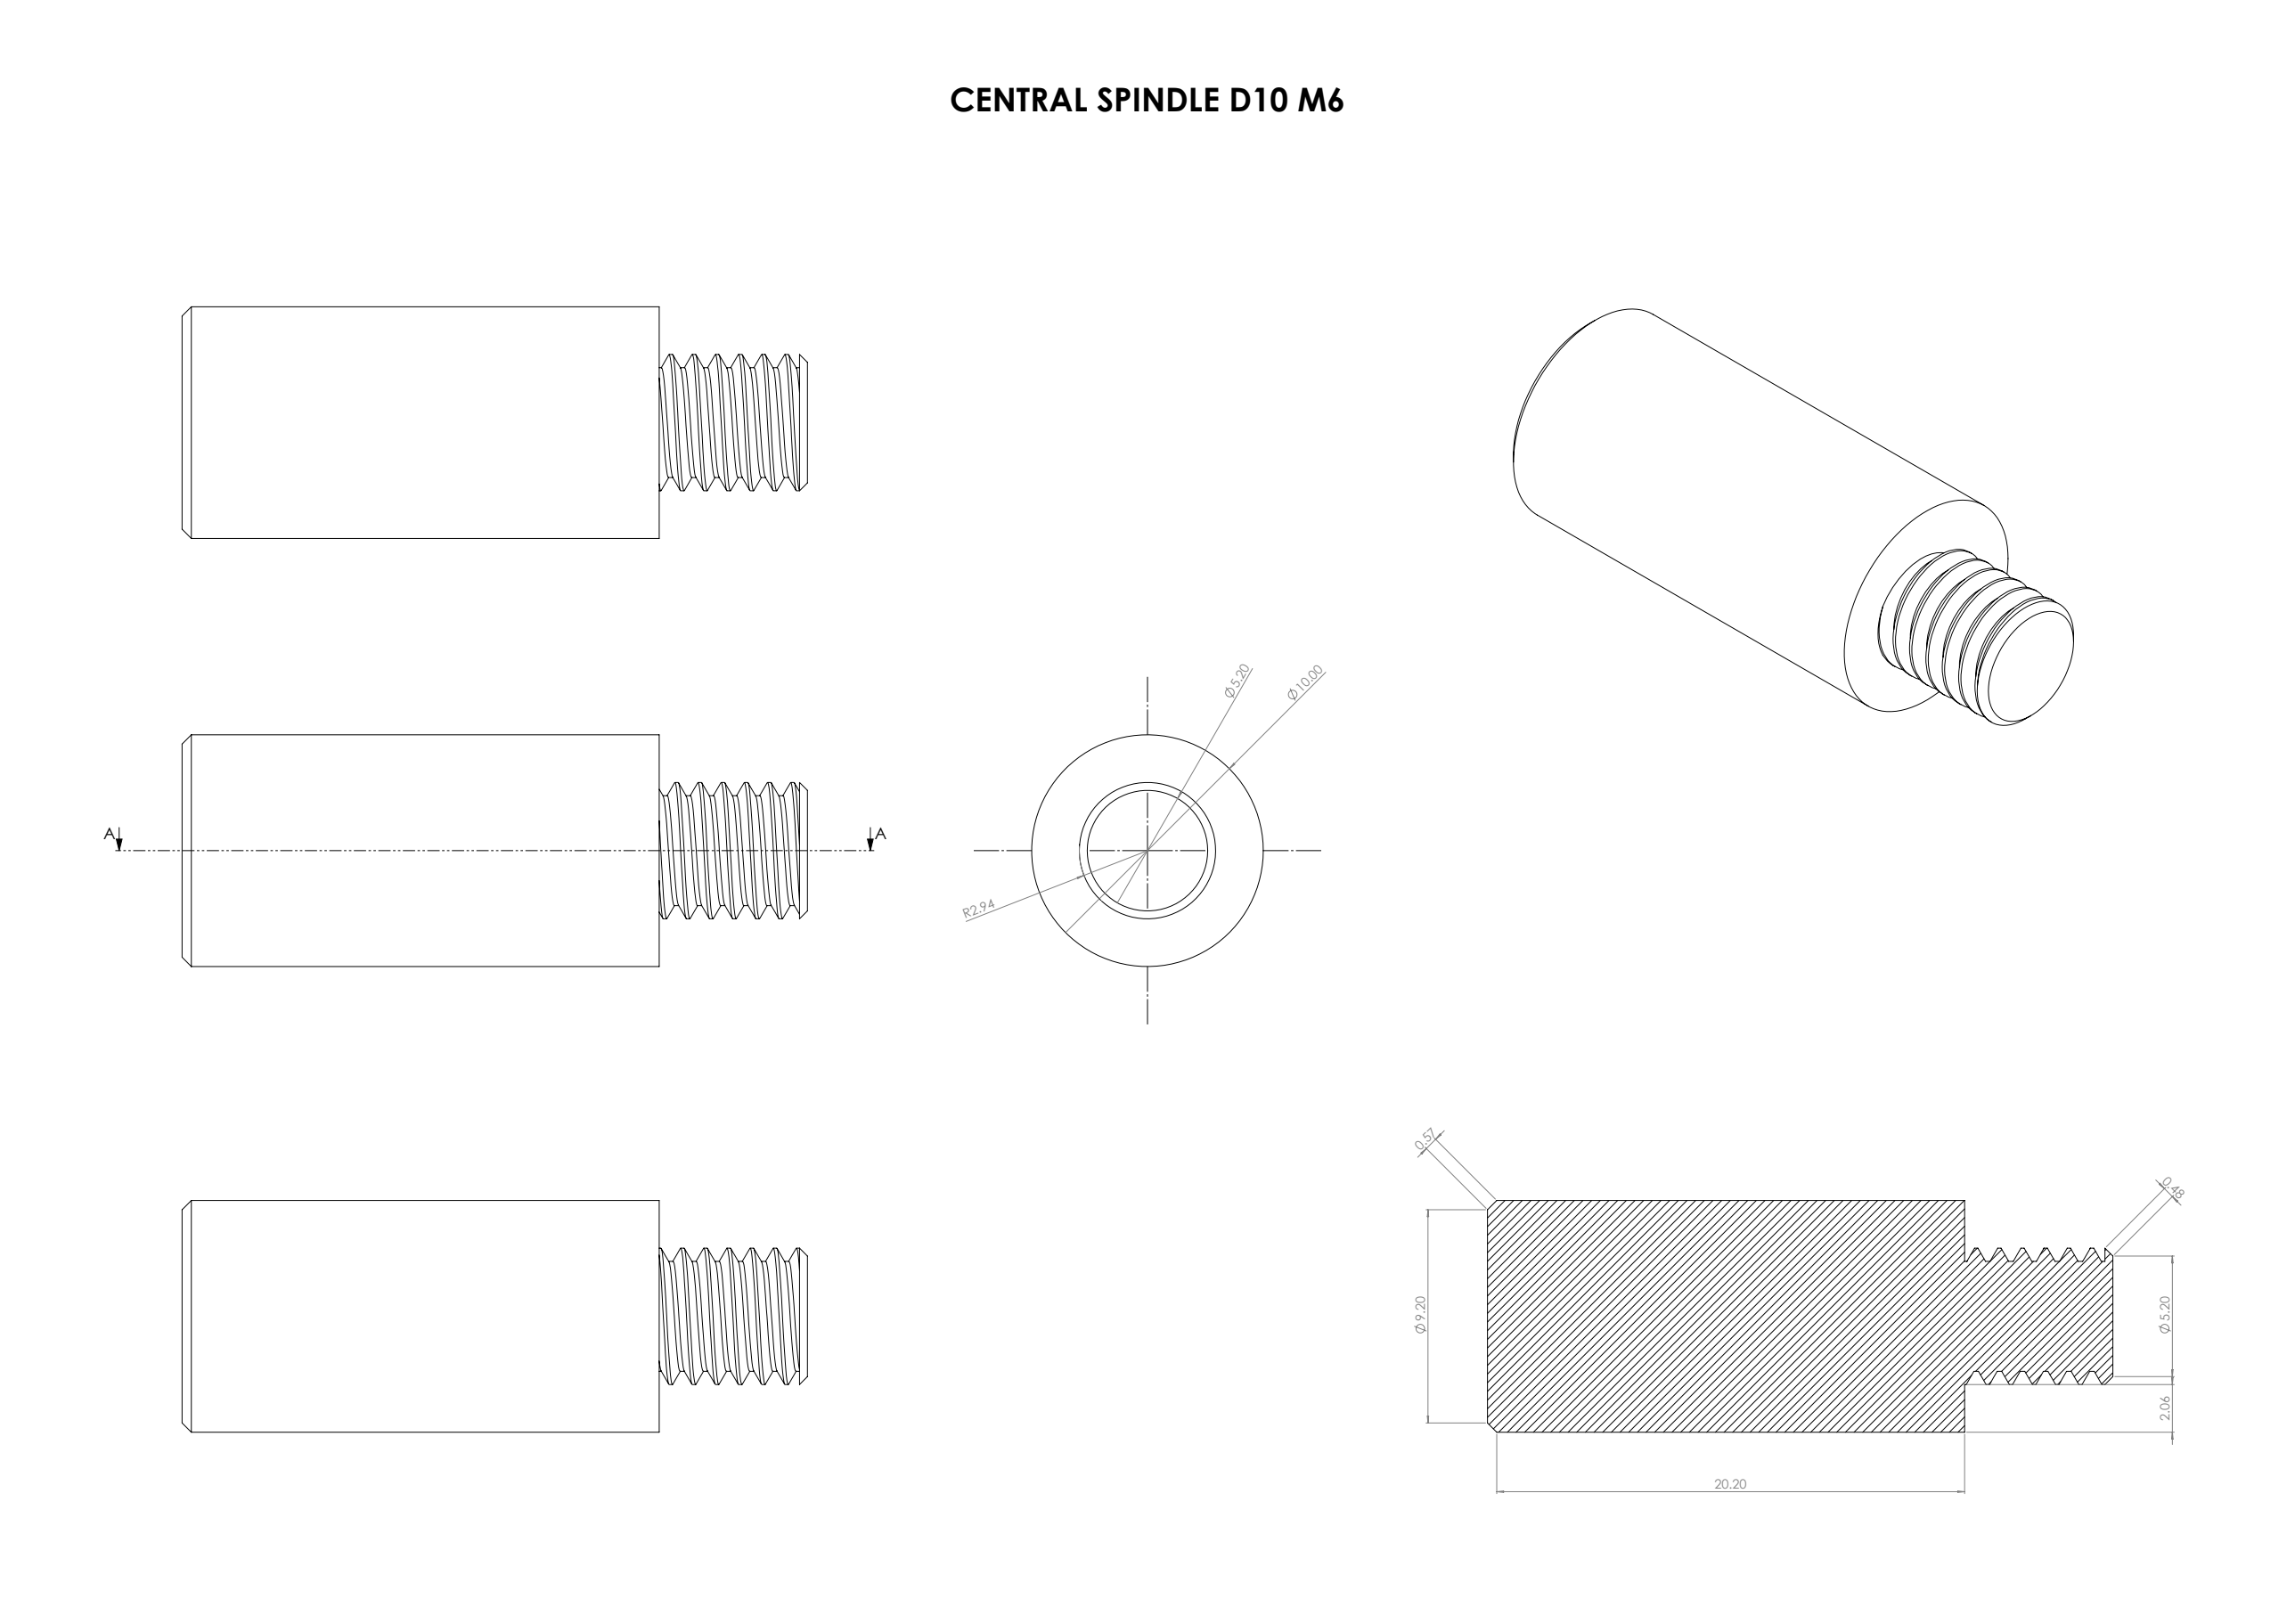
ISO-10303-21;
HEADER;
/* Generated by software containing ST-Developer
 * from STEP Tools, Inc. (www.steptools.com) 
 */

FILE_DESCRIPTION(
/* description */ (''),
/* implementation_level */ '2;1');

FILE_NAME(
/* name */ '04_Central_Spindle_D10_M6.step',
/* time_stamp */ '2026-10-21T02:03:06-07:00',
/* author */ (''),
/* organization */ (''),
/* preprocessor_version */ 'ST-DEVELOPER v20.2',
/* originating_system */ 'Autodesk Translation Framework v15.15.0.0',
/* authorisation */ '');

FILE_SCHEMA (('AUTOMOTIVE_DESIGN { 1 0 10303 214 3 1 1 }'));
ENDSEC;

DATA;
#10=MECHANICAL_DESIGN_GEOMETRIC_PRESENTATION_REPRESENTATION('',(#118),#38528);
#78=B_SPLINE_SURFACE_WITH_KNOTS('',3,3,((#32507,#32508,#32509,#32510,#32511,
#32512,#32513,#32514,#32515,#32516,#32517,#32518,#32519,#32520,#32521,#32522,
#32523,#32524,#32525,#32526,#32527,#32528,#32529,#32530,#32531,#32532,#32533,
#32534,#32535,#32536,#32537,#32538,#32539,#32540,#32541,#32542,#32543,#32544,
#32545,#32546,#32547,#32548,#32549,#32550),(#32551,#32552,#32553,#32554,
#32555,#32556,#32557,#32558,#32559,#32560,#32561,#32562,#32563,#32564,#32565,
#32566,#32567,#32568,#32569,#32570,#32571,#32572,#32573,#32574,#32575,#32576,
#32577,#32578,#32579,#32580,#32581,#32582,#32583,#32584,#32585,#32586,#32587,
#32588,#32589,#32590,#32591,#32592,#32593,#32594),(#32595,#32596,#32597,
#32598,#32599,#32600,#32601,#32602,#32603,#32604,#32605,#32606,#32607,#32608,
#32609,#32610,#32611,#32612,#32613,#32614,#32615,#32616,#32617,#32618,#32619,
#32620,#32621,#32622,#32623,#32624,#32625,#32626,#32627,#32628,#32629,#32630,
#32631,#32632,#32633,#32634,#32635,#32636,#32637,#32638),(#32639,#32640,
#32641,#32642,#32643,#32644,#32645,#32646,#32647,#32648,#32649,#32650,#32651,
#32652,#32653,#32654,#32655,#32656,#32657,#32658,#32659,#32660,#32661,#32662,
#32663,#32664,#32665,#32666,#32667,#32668,#32669,#32670,#32671,#32672,#32673,
#32674,#32675,#32676,#32677,#32678,#32679,#32680,#32681,#32682)),
 .UNSPECIFIED.,.F.,.F.,.F.,(4,4),(4,1,1,1,1,1,1,1,1,1,1,1,1,1,1,1,1,1,1,
1,1,1,1,1,1,1,1,1,1,1,1,1,1,1,1,1,1,1,1,1,1,4),(0.,0.0658467982010769),
(8.30747755240109,9.28631108327433,10.2651446141476,11.2439781450208,12.2228116758941,
13.2016452067673,14.1804787376406,15.1593122685138,16.1381457993871,17.1169793302603,
18.0958128611336,19.0746463920068,20.05347992288,21.0323134537533,22.0111469846265,
22.9899805154998,23.968814046373,24.9476475772463,25.9264811081195,26.9053146389928,
27.884148169866,28.8629817007393,29.8418152316125,30.8206487624858,31.799482293359,
32.7783158242323,33.7571493551055,34.7359828859787,35.714816416852,36.6936499477252,
37.6724834785985,38.6513170094717,39.630150540345,40.6089840712182,41.5878176020915,
42.5666511329647,43.545484663838,44.5243181947112,45.5031517255845,46.4819852564577,
47.460818787331,48.4396523182042),.UNSPECIFIED.);
#79=B_SPLINE_SURFACE_WITH_KNOTS('',3,3,((#32811,#32812,#32813,#32814,#32815,
#32816,#32817,#32818,#32819,#32820,#32821,#32822,#32823,#32824,#32825,#32826,
#32827,#32828,#32829,#32830,#32831,#32832,#32833,#32834,#32835,#32836,#32837,
#32838,#32839,#32840,#32841,#32842,#32843,#32844,#32845,#32846,#32847,#32848,
#32849,#32850,#32851,#32852,#32853,#32854),(#32855,#32856,#32857,#32858,
#32859,#32860,#32861,#32862,#32863,#32864,#32865,#32866,#32867,#32868,#32869,
#32870,#32871,#32872,#32873,#32874,#32875,#32876,#32877,#32878,#32879,#32880,
#32881,#32882,#32883,#32884,#32885,#32886,#32887,#32888,#32889,#32890,#32891,
#32892,#32893,#32894,#32895,#32896,#32897,#32898),(#32899,#32900,#32901,
#32902,#32903,#32904,#32905,#32906,#32907,#32908,#32909,#32910,#32911,#32912,
#32913,#32914,#32915,#32916,#32917,#32918,#32919,#32920,#32921,#32922,#32923,
#32924,#32925,#32926,#32927,#32928,#32929,#32930,#32931,#32932,#32933,#32934,
#32935,#32936,#32937,#32938,#32939,#32940,#32941,#32942),(#32943,#32944,
#32945,#32946,#32947,#32948,#32949,#32950,#32951,#32952,#32953,#32954,#32955,
#32956,#32957,#32958,#32959,#32960,#32961,#32962,#32963,#32964,#32965,#32966,
#32967,#32968,#32969,#32970,#32971,#32972,#32973,#32974,#32975,#32976,#32977,
#32978,#32979,#32980,#32981,#32982,#32983,#32984,#32985,#32986)),
 .UNSPECIFIED.,.F.,.F.,.F.,(4,4),(4,1,1,1,1,1,1,1,1,1,1,1,1,1,1,1,1,1,1,
1,1,1,1,1,1,1,1,1,1,1,1,1,1,1,1,1,1,1,1,1,1,4),(0.,0.0658467982010769),
(11.6150328478183,12.5938663786915,13.5726999095648,14.551533440438,15.5303669713113,
16.5092005021845,17.4880340330578,18.466867563931,19.4457010948043,20.4245346256775,
21.4033681565508,22.382201687424,23.3610352182973,24.3398687491705,25.3187022800437,
26.297535810917,27.2763693417902,28.2552028726635,29.2340364035367,30.21286993441,
31.1917034652832,32.1705369961565,33.1493705270297,34.128204057903,35.1070375887762,
36.0858711196495,37.0647046505227,38.043538181396,39.0223717122692,40.0012052431424,
40.9800387740157,41.9588723048889,42.9377058357622,43.9165393666354,44.8953728975087,
45.8742064283819,46.8530399592552,47.8318734901284,48.8107070210017,49.7895405518749,
50.7683740827482,51.7472076136214),.UNSPECIFIED.);
#94=SHAPE_REPRESENTATION_RELATIONSHIP('SRR','None',#38579,#106);
#106=ADVANCED_BREP_SHAPE_REPRESENTATION('',(#130),#38519);
#118=STYLED_ITEM('',(#38692),#130);
#130=MANIFOLD_SOLID_BREP('Body1',#17075);
#362=CYLINDRICAL_SURFACE('',#18642,2.942);
#363=CYLINDRICAL_SURFACE('',#18644,2.942);
#364=CYLINDRICAL_SURFACE('',#18645,2.942);
#365=CYLINDRICAL_SURFACE('',#18646,2.942);
#366=CYLINDRICAL_SURFACE('',#18647,2.942);
#367=CYLINDRICAL_SURFACE('',#18648,2.942);
#368=CYLINDRICAL_SURFACE('',#18649,2.37175);
#369=CYLINDRICAL_SURFACE('',#18651,2.37175);
#370=CYLINDRICAL_SURFACE('',#18652,2.37175);
#371=CYLINDRICAL_SURFACE('',#18653,2.37175);
#372=CYLINDRICAL_SURFACE('',#18654,2.37175);
#373=CYLINDRICAL_SURFACE('',#18655,2.37175);
#374=CYLINDRICAL_SURFACE('',#18659,2.37175);
#375=CYLINDRICAL_SURFACE('',#18661,2.942);
#376=CYLINDRICAL_SURFACE('',#18667,5.);
#687=B_SPLINE_CURVE_WITH_KNOTS('',3,(#31903,#31904,#31905,#31906,#31907,
#31908,#31909,#31910,#31911,#31912),.UNSPECIFIED.,.F.,.F.,(4,3,3,4),(-4.09293042013066,
-3.91533412349299,-2.93650059261974,-2.06863817490914),.UNSPECIFIED.);
#688=B_SPLINE_CURVE_WITH_KNOTS('',3,(#31915,#31916,#31917,#31918,#31919,
#31920,#31921),.UNSPECIFIED.,.F.,.F.,(4,3,4),(0.,0.978833530873248,1.11730040836829),
 .UNSPECIFIED.);
#689=B_SPLINE_CURVE_WITH_KNOTS('',3,(#31926,#31927,#31928,#31929,#31930,
#31931,#31932,#31933,#31934,#31935,#31936,#31937,#31938,#31939,#31940,#31941,
#31942,#31943,#31944,#31945,#31946,#31947),.UNSPECIFIED.,.F.,.F.,(4,3,3,
3,3,3,3,4),(-10.3761157273103,-9.78833530873246,-8.80950177785921,-7.83066824698597,
-6.85183471611273,-5.87300118523948,-4.89416765436623,-4.09293042013066),
 .UNSPECIFIED.);
#690=B_SPLINE_CURVE_WITH_KNOTS('',3,(#31948,#31949,#31950,#31951,#31952,
#31953,#31954,#31955,#31956,#31957,#31958,#31959,#31960,#31961,#31962,#31963,
#31964,#31965,#31966,#31967,#31968,#31969),.UNSPECIFIED.,.F.,.F.,(4,3,3,
3,3,3,3,4),(1.11730040836829,1.95766706174649,2.93650059261974,3.91533412349299,
4.89416765436624,5.87300118523948,6.85183471611273,7.40048571554788),
 .UNSPECIFIED.);
#691=B_SPLINE_CURVE_WITH_KNOTS('',3,(#31974,#31975,#31976,#31977,#31978,
#31979,#31980,#31981,#31982,#31983,#31984,#31985,#31986,#31987,#31988,#31989,
#31990,#31991,#31992,#31993,#31994,#31995,#31996,#31997,#31998),
 .UNSPECIFIED.,.F.,.F.,(4,3,3,3,3,3,3,3,4),(-16.6593010344898,-16.6401700248452,
-15.6613364939719,-14.6825029630987,-13.7036694322255,-12.7248359013522,
-11.746002370479,-10.7671688396057,-10.3761157273103),.UNSPECIFIED.);
#692=B_SPLINE_CURVE_WITH_KNOTS('',3,(#31999,#32000,#32001,#32002,#32003,
#32004,#32005,#32006,#32007,#32008,#32009,#32010,#32011,#32012,#32013,#32014,
#32015,#32016,#32017,#32018,#32019,#32020),.UNSPECIFIED.,.F.,.F.,(4,3,3,
3,3,3,3,4),(7.40048571554788,7.83066824698597,8.80950177785922,9.78833530873247,
10.7671688396057,11.746002370479,12.7248359013522,13.6836710227275),
 .UNSPECIFIED.);
#693=B_SPLINE_CURVE_WITH_KNOTS('',3,(#32025,#32026,#32027,#32028,#32029,
#32030,#32031,#32032,#32033,#32034,#32035,#32036,#32037,#32038,#32039,#32040,
#32041,#32042,#32043,#32044,#32045,#32046),.UNSPECIFIED.,.F.,.F.,(4,3,3,
3,3,3,3,4),(-22.9424863416694,-22.5131712100847,-21.5343376792114,-20.5555041483382,
-19.5766706174649,-18.5978370865917,-17.6190035557184,-16.6593010344898),
 .UNSPECIFIED.);
#694=B_SPLINE_CURVE_WITH_KNOTS('',3,(#32047,#32048,#32049,#32050,#32051,
#32052,#32053,#32054,#32055,#32056,#32057,#32058,#32059,#32060,#32061,#32062,
#32063,#32064,#32065,#32066,#32067,#32068,#32069,#32070,#32071),
 .UNSPECIFIED.,.F.,.F.,(4,3,3,3,3,3,3,3,4),(13.6836710227275,13.7036694322254,
14.6825029630987,15.6613364939719,16.6401700248452,17.6190035557184,18.5978370865917,
19.5766706174649,19.966856329907),.UNSPECIFIED.);
#695=B_SPLINE_CURVE_WITH_KNOTS('',3,(#32076,#32077,#32078,#32079,#32080,
#32081,#32082,#32083,#32084,#32085,#32086,#32087,#32088,#32089,#32090,#32091,
#32092,#32093,#32094,#32095,#32096,#32097),.UNSPECIFIED.,.F.,.F.,(4,3,3,
3,3,3,3,4),(-29.225671648849,-28.3861723953241,-27.4073388644509,-26.4285053335777,
-25.4496718027044,-24.4708382718312,-23.4920047409579,-22.9424863416694),
 .UNSPECIFIED.);
#696=B_SPLINE_CURVE_WITH_KNOTS('',3,(#32098,#32099,#32100,#32101,#32102,
#32103,#32104,#32105,#32106,#32107,#32108,#32109,#32110,#32111,#32112,#32113,
#32114,#32115,#32116,#32117,#32118,#32119),.UNSPECIFIED.,.F.,.F.,(4,3,3,
3,3,3,3,4),(19.966856329907,20.5555041483382,21.5343376792114,22.5131712100847,
23.4920047409579,24.4708382718312,25.4496718027044,26.2500416370866),
 .UNSPECIFIED.);
#697=B_SPLINE_CURVE_WITH_KNOTS('',3,(#32124,#32125,#32126,#32127,#32128,
#32129,#32130,#32131,#32132,#32133,#32134,#32135,#32136,#32137,#32138,#32139,
#32140,#32141,#32142,#32143,#32144,#32145,#32146,#32147,#32148),
 .UNSPECIFIED.,.F.,.F.,(4,3,3,3,3,3,3,3,4),(-35.5088569560286,-35.2380071114369,
-34.2591735805636,-33.2803400496904,-32.3015065188171,-31.3226729879439,
-30.3438394570706,-29.3650059261974,-29.225671648849),.UNSPECIFIED.);
#698=B_SPLINE_CURVE_WITH_KNOTS('',3,(#32149,#32150,#32151,#32152,#32153,
#32154,#32155,#32156,#32157,#32158,#32159,#32160,#32161,#32162,#32163,#32164,
#32165,#32166,#32167,#32168,#32169,#32170,#32171,#32172,#32173),
 .UNSPECIFIED.,.F.,.F.,(4,3,3,3,3,3,3,3,4),(26.2500416370866,26.4285053335777,
27.4073388644509,28.3861723953241,29.3650059261974,30.3438394570707,31.3226729879439,
32.3015065188171,32.5332269442662),.UNSPECIFIED.);
#699=B_SPLINE_CURVE_WITH_KNOTS('',3,(#32179,#32180,#32181,#32182,#32183,
#32184),.UNSPECIFIED.,.F.,.F.,(4,1,1,4),(47.1238898038469,47.8318734901284,
48.8107070210017,49.6785694387123),.UNSPECIFIED.);
#700=B_SPLINE_CURVE_WITH_KNOTS('',3,(#32187,#32188,#32189,#32190,#32191),
 .UNSPECIFIED.,.F.,.F.,(4,1,4),(47.1238898038469,47.460818787331,48.4396523182042),
 .UNSPECIFIED.);
#701=B_SPLINE_CURVE_WITH_KNOTS('',3,(#32196,#32197,#32198,#32199,#32200,
#32201,#32202,#32203,#32204,#32205,#32206),.UNSPECIFIED.,.F.,.F.,(4,1,1,
1,1,1,1,1,4),(40.8407044966673,40.9800387740157,41.9588723048889,42.9377058357622,
43.9165393666354,44.8953728975087,45.8742064283819,46.8530399592552,47.1238898038469),
 .UNSPECIFIED.);
#702=B_SPLINE_CURVE_WITH_KNOTS('',3,(#32207,#32208,#32209,#32210,#32211,
#32212,#32213,#32214,#32215,#32216),.UNSPECIFIED.,.F.,.F.,(4,1,1,1,1,1,
1,4),(40.8407044966673,41.5878176020915,42.5666511329647,43.545484663838,
44.5243181947112,45.5031517255845,46.4819852564577,47.1238898038469),
 .UNSPECIFIED.);
#703=B_SPLINE_CURVE_WITH_KNOTS('',3,(#32221,#32222,#32223,#32224,#32225,
#32226,#32227,#32228,#32229,#32230),.UNSPECIFIED.,.F.,.F.,(4,1,1,1,1,1,
1,4),(34.5575191894877,35.1070375887762,36.0858711196495,37.0647046505227,
38.043538181396,39.0223717122692,40.0012052431424,40.8407044966673),
 .UNSPECIFIED.);
#704=B_SPLINE_CURVE_WITH_KNOTS('',3,(#32231,#32232,#32233,#32234,#32235,
#32236,#32237,#32238,#32239,#32240,#32241),.UNSPECIFIED.,.F.,.F.,(4,1,1,
1,1,1,1,1,4),(34.5575191894877,34.7359828859787,35.714816416852,36.6936499477252,
37.6724834785985,38.6513170094717,39.630150540345,40.6089840712182,40.8407044966673),
 .UNSPECIFIED.);
#705=B_SPLINE_CURVE_WITH_KNOTS('',3,(#32246,#32247,#32248,#32249,#32250,
#32251,#32252,#32253,#32254,#32255),.UNSPECIFIED.,.F.,.F.,(4,1,1,1,1,1,
1,4),(28.2743338823081,29.2340364035367,30.21286993441,31.1917034652832,
32.1705369961565,33.1493705270297,34.128204057903,34.5575191894877),
 .UNSPECIFIED.);
#706=B_SPLINE_CURVE_WITH_KNOTS('',3,(#32256,#32257,#32258,#32259,#32260,
#32261,#32262,#32263,#32264,#32265),.UNSPECIFIED.,.F.,.F.,(4,1,1,1,1,1,
1,4),(28.2743338823081,28.8629817007393,29.8418152316125,30.8206487624858,
31.799482293359,32.7783158242323,33.7571493551055,34.5575191894877),
 .UNSPECIFIED.);
#707=B_SPLINE_CURVE_WITH_KNOTS('',3,(#32270,#32271,#32272,#32273,#32274,
#32275,#32276,#32277,#32278,#32279,#32280),.UNSPECIFIED.,.F.,.F.,(4,1,1,
1,1,1,1,1,4),(21.9911485751285,22.382201687424,23.3610352182973,24.3398687491705,
25.3187022800437,26.297535810917,27.2763693417902,28.2552028726635,28.2743338823081),
 .UNSPECIFIED.);
#708=B_SPLINE_CURVE_WITH_KNOTS('',3,(#32281,#32282,#32283,#32284,#32285,
#32286,#32287,#32288,#32289,#32290,#32291),.UNSPECIFIED.,.F.,.F.,(4,1,1,
1,1,1,1,1,4),(21.9911485751285,22.0111469846265,22.9899805154998,23.968814046373,
24.9476475772463,25.9264811081195,26.9053146389928,27.884148169866,28.2743338823081),
 .UNSPECIFIED.);
#709=B_SPLINE_CURVE_WITH_KNOTS('',3,(#32296,#32297,#32298,#32299,#32300,
#32301,#32302,#32303,#32304,#32305),.UNSPECIFIED.,.F.,.F.,(4,1,1,1,1,1,
1,4),(15.7079632679489,16.5092005021845,17.4880340330578,18.466867563931,
19.4457010948043,20.4245346256775,21.4033681565508,21.9911485751285),
 .UNSPECIFIED.);
#710=B_SPLINE_CURVE_WITH_KNOTS('',3,(#32306,#32307,#32308,#32309,#32310,
#32311,#32312,#32313,#32314,#32315),.UNSPECIFIED.,.F.,.F.,(4,1,1,1,1,1,
1,4),(15.7079632679489,16.1381457993871,17.1169793302603,18.0958128611336,
19.0746463920068,20.05347992288,21.0323134537533,21.9911485751285),
 .UNSPECIFIED.);
#711=B_SPLINE_CURVE_WITH_KNOTS('',3,(#32318,#32319,#32320,#32321,#32322,
#32323,#32324,#32325,#32326,#32327,#32328,#32329,#32330,#32331,#32332,#32333,
#32334,#32335,#32336,#32337,#32338,#32339,#32340,#32341,#32342,#32343,#32344,
#32345,#32346,#32347,#32348,#32349,#32350,#32351,#32352,#32353,#32354,#32355,
#32356,#32357,#32358,#32359,#32360,#32361,#32362,#32363,#32364,#32365,#32366,
#32367,#32368,#32369,#32370,#32371,#32372,#32373,#32374,#32375,#32376,#32377,
#32378,#32379,#32380,#32381,#32382,#32383,#32384,#32385,#32386,#32387,#32388,
#32389,#32390,#32391,#32392,#32393,#32394,#32395,#32396,#32397,#32398,#32399,
#32400,#32401,#32402,#32403,#32404,#32405),.UNSPECIFIED.,.F.,.F.,(4,3,3,
3,3,3,3,3,3,3,3,3,3,3,3,3,3,3,3,3,3,3,3,3,3,3,3,3,3,4),(-0.555272788399365,
-0.52846767863439,-0.503594637637908,-0.491620530364568,-0.486548771256777,
-0.46038777702908,-0.437496907079845,-0.430089856089214,-0.425283241489225,
-0.420739109591328,-0.394172021992522,-0.367149700387639,-0.344677479649528,
-0.327654949218049,-0.322163644667068,-0.294255571126051,-0.277260817435197,
-0.250234732978329,-0.234595062167183,-0.223439460304812,-0.217840497360261,
-0.189937324364723,-0.161486698536973,-0.132774069185219,-0.116177310537067,
-0.111767824711868,-0.0823316934096331,-0.0527876353241155,-0.0237740161581124,
0.),.UNSPECIFIED.);
#712=B_SPLINE_CURVE_WITH_KNOTS('',3,(#32410,#32411,#32412,#32413,#32414,
#32415,#32416,#32417,#32418,#32419,#32420,#32421,#32422,#32423,#32424,#32425,
#32426,#32427,#32428,#32429,#32430,#32431,#32432,#32433,#32434,#32435,#32436,
#32437,#32438,#32439,#32440,#32441,#32442,#32443,#32444,#32445,#32446,#32447,
#32448,#32449,#32450,#32451,#32452,#32453,#32454,#32455,#32456,#32457,#32458,
#32459,#32460,#32461,#32462,#32463,#32464,#32465,#32466,#32467,#32468,#32469,
#32470,#32471,#32472,#32473,#32474,#32475,#32476,#32477,#32478,#32479,#32480,
#32481,#32482,#32483,#32484,#32485,#32486,#32487,#32488,#32489,#32490,#32491,
#32492,#32493,#32494,#32495,#32496,#32497,#32498,#32499,#32500,#32501,#32502,
#32503,#32504,#32505,#32506),.UNSPECIFIED.,.F.,.F.,(4,3,3,3,3,3,3,3,3,3,
3,3,3,3,3,3,3,3,3,3,3,3,3,3,3,3,3,3,3,3,3,3,4),(-0.552745378375028,-0.524051566310883,
-0.520210139258523,-0.490737208406128,-0.482065926984848,-0.476361701638012,
-0.470495789890482,-0.441459967293392,-0.417194500231044,-0.406393530772314,
-0.401030964911425,-0.39612764238736,-0.36782565203914,-0.339770953176154,
-0.316662272580769,-0.29933076213423,-0.294967834876196,-0.290936046393434,
-0.26412806323215,-0.247336230794614,-0.219938258183661,-0.192445975910703,
-0.188229859720074,-0.16160728097907,-0.135010228556239,-0.108826952648143,
-0.0998939422463041,-0.0942306910950506,-0.0901865085424749,-0.0646366135836345,
-0.0394819043305994,-0.0151075305849294,0.),.UNSPECIFIED.);
#713=B_SPLINE_CURVE_WITH_KNOTS('',3,(#32683,#32684,#32685,#32686,#32687,
#32688,#32689,#32690,#32691,#32692,#32693,#32694,#32695,#32696,#32697,#32698,
#32699,#32700,#32701),.UNSPECIFIED.,.F.,.F.,(4,3,3,3,3,3,4),(32.5332269442662,
33.2803400496904,34.2591735805636,35.2380071114369,36.2168406423101,37.1956741731834,
38.063536590894),.UNSPECIFIED.);
#714=B_SPLINE_CURVE_WITH_KNOTS('',3,(#32703,#32704,#32705,#32706,#32707,
#32708,#32709,#32710,#32711,#32712,#32713,#32714,#32715,#32716,#32717,#32718,
#32719,#32720,#32721,#32722,#32723,#32724,#32725,#32726,#32727,#32728,#32729,
#32730,#32731,#32732,#32733,#32734,#32735,#32736,#32737,#32738,#32739,#32740,
#32741,#32742,#32743,#32744,#32745,#32746,#32747,#32748,#32749,#32750,#32751,
#32752,#32753,#32754,#32755,#32756,#32757,#32758,#32759,#32760,#32761,#32762,
#32763,#32764,#32765,#32766,#32767,#32768,#32769,#32770,#32771,#32772,#32773,
#32774,#32775,#32776,#32777,#32778,#32779,#32780,#32781,#32782,#32783,#32784,
#32785,#32786,#32787,#32788,#32789,#32790),.UNSPECIFIED.,.F.,.F.,(4,3,3,
3,3,3,3,3,3,3,3,3,3,3,3,3,3,3,3,3,3,3,3,3,3,3,3,3,3,4),(-0.555272788399382,
-0.528467678634411,-0.503594611950225,-0.491620530448705,-0.486548768208902,
-0.460387774362191,-0.437496904746319,-0.430089843892791,-0.42528335746406,
-0.420739137835661,-0.394172035990758,-0.367149711920146,-0.344677488298913,
-0.327654967351694,-0.322163642962578,-0.29425557103191,-0.277260817435213,
-0.250234719828173,-0.234595049838912,-0.223439458719702,-0.217840498614478,
-0.18993731124497,-0.16148667063061,-0.132774036478808,-0.116177281918957,
-0.111767791045449,-0.0823316491114678,-0.0527875952217257,-0.0237740134204675,
0.),.UNSPECIFIED.);
#715=B_SPLINE_CURVE_WITH_KNOTS('',3,(#32791,#32792,#32793,#32794,#32795,
#32796,#32797,#32798,#32799),.UNSPECIFIED.,.F.,.F.,(4,1,1,1,1,1,4),(10.3761157273102,
11.2439781450208,12.2228116758941,13.2016452067673,14.1804787376406,15.1593122685138,
15.7079632679489),.UNSPECIFIED.);
#716=B_SPLINE_CURVE_WITH_KNOTS('',3,(#32803,#32804,#32805,#32806,#32807,
#32808,#32809,#32810),.UNSPECIFIED.,.F.,.F.,(4,1,1,1,1,4),(11.6150328478183,
12.5938663786915,13.5726999095648,14.551533440438,15.5303669713113,15.7079632679489),
 .UNSPECIFIED.);
#717=B_SPLINE_CURVE_WITH_KNOTS('',3,(#32987,#32988,#32989,#32990,#32991,
#32992,#32993,#32994,#32995,#32996,#32997,#32998,#32999,#33000,#33001,#33002,
#33003,#33004,#33005,#33006,#33007,#33008,#33009,#33010,#33011,#33012,#33013,
#33014,#33015,#33016,#33017,#33018,#33019,#33020,#33021,#33022,#33023,#33024,
#33025,#33026,#33027,#33028,#33029,#33030,#33031,#33032,#33033,#33034,#33035,
#33036,#33037,#33038,#33039,#33040,#33041,#33042,#33043,#33044,#33045,#33046,
#33047,#33048,#33049,#33050,#33051,#33052,#33053,#33054,#33055,#33056,#33057,
#33058,#33059,#33060,#33061,#33062,#33063,#33064,#33065,#33066,#33067,#33068,
#33069,#33070,#33071,#33072,#33073,#33074,#33075,#33076,#33077,#33078,#33079,
#33080,#33081,#33082,#33083),.UNSPECIFIED.,.F.,.F.,(4,3,3,3,3,3,3,3,3,3,
3,3,3,3,3,3,3,3,3,3,3,3,3,3,3,3,3,3,3,3,3,3,4),(-0.552745378375046,-0.524051576025582,
-0.520210139258547,-0.490737207720614,-0.482065932922306,-0.476361784855821,
-0.470495811804092,-0.441459989540148,-0.417194519696956,-0.406393563117289,
-0.401031128507146,-0.396127678339415,-0.367825690719443,-0.339771006600577,
-0.316662312649086,-0.299330792185467,-0.294967891446945,-0.290936172565379,
-0.264128215008968,-0.247336230794613,-0.219938271840149,-0.192445987860131,
-0.188229859754739,-0.161607289273899,-0.135010221728073,-0.108826909841477,
-0.0998938267520413,-0.0942311920104265,-0.0901865995336686,-0.0646366752402619,
-0.0394819229126391,-0.0151074961268136,0.),.UNSPECIFIED.);
#718=B_SPLINE_CURVE_WITH_KNOTS('',3,(#33084,#33085,#33086,#33087,#33088,
#33089,#33090,#33091,#33092,#33093,#33094,#33095,#33096,#33097,#33098,#33099),
 .UNSPECIFIED.,.F.,.F.,(4,3,3,3,3,4),(-40.1321747658031,-39.1533412349299,
-38.1745077040566,-37.1956741731834,-36.2168406423101,-35.5088569560286),
 .UNSPECIFIED.);
#1029=CONICAL_SURFACE('',#18665,4.8,0.785398163397449);
#1030=CONICAL_SURFACE('',#18670,2.8,0.785398163397453);
#1465=FACE_BOUND('',#4058,.T.);
#2150=CIRCLE('',#18643,2.942);
#2151=CIRCLE('',#18650,2.37175);
#2152=CIRCLE('',#18657,2.942);
#2153=CIRCLE('',#18658,2.942);
#2154=CIRCLE('',#18660,2.37175);
#2155=CIRCLE('',#18662,2.942);
#2156=CIRCLE('',#18664,4.6);
#2157=CIRCLE('',#18666,5.);
#2158=CIRCLE('',#18668,5.);
#2159=CIRCLE('',#18671,2.6);
#3021=FACE_OUTER_BOUND('',#4037,.T.);
#3022=FACE_OUTER_BOUND('',#4038,.T.);
#3023=FACE_OUTER_BOUND('',#4039,.T.);
#3024=FACE_OUTER_BOUND('',#4040,.T.);
#3025=FACE_OUTER_BOUND('',#4041,.T.);
#3026=FACE_OUTER_BOUND('',#4042,.T.);
#3027=FACE_OUTER_BOUND('',#4043,.T.);
#3028=FACE_OUTER_BOUND('',#4044,.T.);
#3029=FACE_OUTER_BOUND('',#4045,.T.);
#3030=FACE_OUTER_BOUND('',#4046,.T.);
#3031=FACE_OUTER_BOUND('',#4047,.T.);
#3032=FACE_OUTER_BOUND('',#4048,.T.);
#3033=FACE_OUTER_BOUND('',#4049,.T.);
#3034=FACE_OUTER_BOUND('',#4050,.T.);
#3035=FACE_OUTER_BOUND('',#4051,.T.);
#3036=FACE_OUTER_BOUND('',#4052,.T.);
#3037=FACE_OUTER_BOUND('',#4053,.T.);
#3038=FACE_OUTER_BOUND('',#4054,.T.);
#3039=FACE_OUTER_BOUND('',#4055,.T.);
#3040=FACE_OUTER_BOUND('',#4056,.T.);
#3041=FACE_OUTER_BOUND('',#4057,.T.);
#3042=FACE_OUTER_BOUND('',#4059,.T.);
#3043=FACE_OUTER_BOUND('',#4060,.T.);
#4037=EDGE_LOOP('',(#14365,#14366,#14367,#14368));
#4038=EDGE_LOOP('',(#14369,#14370,#14371,#14372));
#4039=EDGE_LOOP('',(#14373,#14374,#14375,#14376));
#4040=EDGE_LOOP('',(#14377,#14378,#14379,#14380));
#4041=EDGE_LOOP('',(#14381,#14382,#14383,#14384));
#4042=EDGE_LOOP('',(#14385,#14386,#14387,#14388));
#4043=EDGE_LOOP('',(#14389,#14390,#14391,#14392));
#4044=EDGE_LOOP('',(#14393,#14394,#14395,#14396));
#4045=EDGE_LOOP('',(#14397,#14398,#14399,#14400));
#4046=EDGE_LOOP('',(#14401,#14402,#14403,#14404));
#4047=EDGE_LOOP('',(#14405,#14406,#14407,#14408));
#4048=EDGE_LOOP('',(#14409,#14410,#14411,#14412));
#4049=EDGE_LOOP('',(#14413,#14414,#14415,#14416,#14417));
#4050=EDGE_LOOP('',(#14418,#14419,#14420,#14421,#14422,#14423,#14424,#14425,
#14426,#14427,#14428,#14429,#14430,#14431,#14432,#14433));
#4051=EDGE_LOOP('',(#14434,#14435,#14436,#14437));
#4052=EDGE_LOOP('',(#14438,#14439,#14440,#14441,#14442,#14443,#14444,#14445,
#14446,#14447,#14448,#14449,#14450,#14451,#14452,#14453));
#4053=EDGE_LOOP('',(#14454,#14455,#14456,#14457));
#4054=EDGE_LOOP('',(#14458));
#4055=EDGE_LOOP('',(#14459,#14460,#14461,#14462));
#4056=EDGE_LOOP('',(#14463,#14464,#14465,#14466));
#4057=EDGE_LOOP('',(#14467));
#4058=EDGE_LOOP('',(#14468,#14469,#14470,#14471));
#4059=EDGE_LOOP('',(#14472,#14473,#14474,#14475,#14476,#14477));
#4060=EDGE_LOOP('',(#14478));
#5004=LINE('',#31901,#5979);
#5005=LINE('',#31925,#5980);
#5006=LINE('',#31973,#5981);
#5007=LINE('',#32024,#5982);
#5008=LINE('',#32075,#5983);
#5009=LINE('',#32123,#5984);
#5010=LINE('',#32177,#5985);
#5011=LINE('',#32195,#5986);
#5012=LINE('',#32220,#5987);
#5013=LINE('',#32245,#5988);
#5014=LINE('',#32269,#5989);
#5015=LINE('',#32295,#5990);
#5016=LINE('',#33108,#5991);
#5017=LINE('',#33112,#5992);
#5018=LINE('',#33117,#5993);
#5979=VECTOR('',#22590,3.);
#5980=VECTOR('',#22595,3.);
#5981=VECTOR('',#22598,3.);
#5982=VECTOR('',#22601,3.);
#5983=VECTOR('',#22604,3.);
#5984=VECTOR('',#22607,3.);
#5985=VECTOR('',#22610,2.37175);
#5986=VECTOR('',#22615,2.37175);
#5987=VECTOR('',#22618,2.37175);
#5988=VECTOR('',#22621,2.37175);
#5989=VECTOR('',#22624,2.37175);
#5990=VECTOR('',#22627,2.37175);
#5991=VECTOR('',#22650,4.8);
#5992=VECTOR('',#22655,5.);
#5993=VECTOR('',#22662,2.8);
#7474=VERTEX_POINT('',#31899);
#7475=VERTEX_POINT('',#31900);
#7476=VERTEX_POINT('',#31902);
#7477=VERTEX_POINT('',#31913);
#7478=VERTEX_POINT('',#31923);
#7479=VERTEX_POINT('',#31924);
#7480=VERTEX_POINT('',#31971);
#7481=VERTEX_POINT('',#31972);
#7482=VERTEX_POINT('',#32022);
#7483=VERTEX_POINT('',#32023);
#7484=VERTEX_POINT('',#32073);
#7485=VERTEX_POINT('',#32074);
#7486=VERTEX_POINT('',#32121);
#7487=VERTEX_POINT('',#32122);
#7488=VERTEX_POINT('',#32175);
#7489=VERTEX_POINT('',#32176);
#7490=VERTEX_POINT('',#32178);
#7491=VERTEX_POINT('',#32185);
#7492=VERTEX_POINT('',#32193);
#7493=VERTEX_POINT('',#32194);
#7494=VERTEX_POINT('',#32218);
#7495=VERTEX_POINT('',#32219);
#7496=VERTEX_POINT('',#32243);
#7497=VERTEX_POINT('',#32244);
#7498=VERTEX_POINT('',#32267);
#7499=VERTEX_POINT('',#32268);
#7500=VERTEX_POINT('',#32293);
#7501=VERTEX_POINT('',#32294);
#7502=VERTEX_POINT('',#32317);
#7503=VERTEX_POINT('',#32406);
#7504=VERTEX_POINT('',#32408);
#7505=VERTEX_POINT('',#32702);
#7506=VERTEX_POINT('',#32801);
#7507=VERTEX_POINT('',#33103);
#7508=VERTEX_POINT('',#33106);
#7509=VERTEX_POINT('',#33110);
#7510=VERTEX_POINT('',#33115);
#9834=EDGE_CURVE('',#7474,#7475,#5004,.T.);
#9835=EDGE_CURVE('',#7474,#7476,#687,.T.);
#9836=EDGE_CURVE('',#7476,#7477,#2150,.F.);
#9837=EDGE_CURVE('',#7477,#7475,#688,.T.);
#9838=EDGE_CURVE('',#7478,#7479,#5005,.T.);
#9839=EDGE_CURVE('',#7478,#7474,#689,.T.);
#9840=EDGE_CURVE('',#7475,#7479,#690,.T.);
#9841=EDGE_CURVE('',#7480,#7481,#5006,.T.);
#9842=EDGE_CURVE('',#7480,#7478,#691,.T.);
#9843=EDGE_CURVE('',#7479,#7481,#692,.T.);
#9844=EDGE_CURVE('',#7482,#7483,#5007,.T.);
#9845=EDGE_CURVE('',#7482,#7480,#693,.T.);
#9846=EDGE_CURVE('',#7481,#7483,#694,.T.);
#9847=EDGE_CURVE('',#7484,#7485,#5008,.T.);
#9848=EDGE_CURVE('',#7484,#7482,#695,.T.);
#9849=EDGE_CURVE('',#7483,#7485,#696,.T.);
#9850=EDGE_CURVE('',#7486,#7487,#5009,.T.);
#9851=EDGE_CURVE('',#7486,#7484,#697,.T.);
#9852=EDGE_CURVE('',#7485,#7487,#698,.T.);
#9853=EDGE_CURVE('',#7488,#7489,#5010,.T.);
#9854=EDGE_CURVE('',#7488,#7490,#699,.T.);
#9855=EDGE_CURVE('',#7491,#7490,#2151,.T.);
#9856=EDGE_CURVE('',#7489,#7491,#700,.T.);
#9857=EDGE_CURVE('',#7492,#7493,#5011,.T.);
#9858=EDGE_CURVE('',#7492,#7488,#701,.T.);
#9859=EDGE_CURVE('',#7493,#7489,#702,.T.);
#9860=EDGE_CURVE('',#7494,#7495,#5012,.T.);
#9861=EDGE_CURVE('',#7494,#7492,#703,.T.);
#9862=EDGE_CURVE('',#7495,#7493,#704,.T.);
#9863=EDGE_CURVE('',#7496,#7497,#5013,.T.);
#9864=EDGE_CURVE('',#7496,#7494,#705,.T.);
#9865=EDGE_CURVE('',#7497,#7495,#706,.T.);
#9866=EDGE_CURVE('',#7498,#7499,#5014,.T.);
#9867=EDGE_CURVE('',#7498,#7496,#707,.T.);
#9868=EDGE_CURVE('',#7499,#7497,#708,.T.);
#9869=EDGE_CURVE('',#7500,#7501,#5015,.T.);
#9870=EDGE_CURVE('',#7500,#7498,#709,.T.);
#9871=EDGE_CURVE('',#7501,#7499,#710,.T.);
#9872=EDGE_CURVE('',#7490,#7502,#711,.T.);
#9873=EDGE_CURVE('',#7503,#7502,#2152,.F.);
#9874=EDGE_CURVE('',#7504,#7503,#2153,.F.);
#9875=EDGE_CURVE('',#7504,#7491,#712,.T.);
#9876=EDGE_CURVE('',#7487,#7504,#713,.T.);
#9877=EDGE_CURVE('',#7505,#7477,#714,.T.);
#9878=EDGE_CURVE('',#7505,#7501,#715,.T.);
#9879=EDGE_CURVE('',#7506,#7505,#2154,.T.);
#9880=EDGE_CURVE('',#7506,#7500,#716,.T.);
#9881=EDGE_CURVE('',#7476,#7506,#717,.T.);
#9882=EDGE_CURVE('',#7502,#7486,#718,.T.);
#9883=EDGE_CURVE('',#7502,#7504,#2155,.F.);
#9884=EDGE_CURVE('',#7507,#7507,#2156,.T.);
#9885=EDGE_CURVE('',#7508,#7508,#2157,.T.);
#9886=EDGE_CURVE('',#7508,#7507,#5016,.T.);
#9887=EDGE_CURVE('',#7509,#7509,#2158,.T.);
#9888=EDGE_CURVE('',#7509,#7508,#5017,.T.);
#9889=EDGE_CURVE('',#7510,#7510,#2159,.T.);
#9890=EDGE_CURVE('',#7510,#7503,#5018,.T.);
#14365=ORIENTED_EDGE('',*,*,#9834,.F.);
#14366=ORIENTED_EDGE('',*,*,#9835,.T.);
#14367=ORIENTED_EDGE('',*,*,#9836,.T.);
#14368=ORIENTED_EDGE('',*,*,#9837,.T.);
#14369=ORIENTED_EDGE('',*,*,#9838,.F.);
#14370=ORIENTED_EDGE('',*,*,#9839,.T.);
#14371=ORIENTED_EDGE('',*,*,#9834,.T.);
#14372=ORIENTED_EDGE('',*,*,#9840,.T.);
#14373=ORIENTED_EDGE('',*,*,#9841,.F.);
#14374=ORIENTED_EDGE('',*,*,#9842,.T.);
#14375=ORIENTED_EDGE('',*,*,#9838,.T.);
#14376=ORIENTED_EDGE('',*,*,#9843,.T.);
#14377=ORIENTED_EDGE('',*,*,#9844,.F.);
#14378=ORIENTED_EDGE('',*,*,#9845,.T.);
#14379=ORIENTED_EDGE('',*,*,#9841,.T.);
#14380=ORIENTED_EDGE('',*,*,#9846,.T.);
#14381=ORIENTED_EDGE('',*,*,#9847,.F.);
#14382=ORIENTED_EDGE('',*,*,#9848,.T.);
#14383=ORIENTED_EDGE('',*,*,#9844,.T.);
#14384=ORIENTED_EDGE('',*,*,#9849,.T.);
#14385=ORIENTED_EDGE('',*,*,#9850,.F.);
#14386=ORIENTED_EDGE('',*,*,#9851,.T.);
#14387=ORIENTED_EDGE('',*,*,#9847,.T.);
#14388=ORIENTED_EDGE('',*,*,#9852,.T.);
#14389=ORIENTED_EDGE('',*,*,#9853,.F.);
#14390=ORIENTED_EDGE('',*,*,#9854,.T.);
#14391=ORIENTED_EDGE('',*,*,#9855,.F.);
#14392=ORIENTED_EDGE('',*,*,#9856,.F.);
#14393=ORIENTED_EDGE('',*,*,#9857,.F.);
#14394=ORIENTED_EDGE('',*,*,#9858,.T.);
#14395=ORIENTED_EDGE('',*,*,#9853,.T.);
#14396=ORIENTED_EDGE('',*,*,#9859,.F.);
#14397=ORIENTED_EDGE('',*,*,#9860,.F.);
#14398=ORIENTED_EDGE('',*,*,#9861,.T.);
#14399=ORIENTED_EDGE('',*,*,#9857,.T.);
#14400=ORIENTED_EDGE('',*,*,#9862,.F.);
#14401=ORIENTED_EDGE('',*,*,#9863,.F.);
#14402=ORIENTED_EDGE('',*,*,#9864,.T.);
#14403=ORIENTED_EDGE('',*,*,#9860,.T.);
#14404=ORIENTED_EDGE('',*,*,#9865,.F.);
#14405=ORIENTED_EDGE('',*,*,#9866,.F.);
#14406=ORIENTED_EDGE('',*,*,#9867,.T.);
#14407=ORIENTED_EDGE('',*,*,#9863,.T.);
#14408=ORIENTED_EDGE('',*,*,#9868,.F.);
#14409=ORIENTED_EDGE('',*,*,#9869,.F.);
#14410=ORIENTED_EDGE('',*,*,#9870,.T.);
#14411=ORIENTED_EDGE('',*,*,#9866,.T.);
#14412=ORIENTED_EDGE('',*,*,#9871,.F.);
#14413=ORIENTED_EDGE('',*,*,#9855,.T.);
#14414=ORIENTED_EDGE('',*,*,#9872,.T.);
#14415=ORIENTED_EDGE('',*,*,#9873,.F.);
#14416=ORIENTED_EDGE('',*,*,#9874,.F.);
#14417=ORIENTED_EDGE('',*,*,#9875,.T.);
#14418=ORIENTED_EDGE('',*,*,#9875,.F.);
#14419=ORIENTED_EDGE('',*,*,#9876,.F.);
#14420=ORIENTED_EDGE('',*,*,#9852,.F.);
#14421=ORIENTED_EDGE('',*,*,#9849,.F.);
#14422=ORIENTED_EDGE('',*,*,#9846,.F.);
#14423=ORIENTED_EDGE('',*,*,#9843,.F.);
#14424=ORIENTED_EDGE('',*,*,#9840,.F.);
#14425=ORIENTED_EDGE('',*,*,#9837,.F.);
#14426=ORIENTED_EDGE('',*,*,#9877,.F.);
#14427=ORIENTED_EDGE('',*,*,#9878,.T.);
#14428=ORIENTED_EDGE('',*,*,#9871,.T.);
#14429=ORIENTED_EDGE('',*,*,#9868,.T.);
#14430=ORIENTED_EDGE('',*,*,#9865,.T.);
#14431=ORIENTED_EDGE('',*,*,#9862,.T.);
#14432=ORIENTED_EDGE('',*,*,#9859,.T.);
#14433=ORIENTED_EDGE('',*,*,#9856,.T.);
#14434=ORIENTED_EDGE('',*,*,#9869,.T.);
#14435=ORIENTED_EDGE('',*,*,#9878,.F.);
#14436=ORIENTED_EDGE('',*,*,#9879,.F.);
#14437=ORIENTED_EDGE('',*,*,#9880,.T.);
#14438=ORIENTED_EDGE('',*,*,#9872,.F.);
#14439=ORIENTED_EDGE('',*,*,#9854,.F.);
#14440=ORIENTED_EDGE('',*,*,#9858,.F.);
#14441=ORIENTED_EDGE('',*,*,#9861,.F.);
#14442=ORIENTED_EDGE('',*,*,#9864,.F.);
#14443=ORIENTED_EDGE('',*,*,#9867,.F.);
#14444=ORIENTED_EDGE('',*,*,#9870,.F.);
#14445=ORIENTED_EDGE('',*,*,#9880,.F.);
#14446=ORIENTED_EDGE('',*,*,#9881,.F.);
#14447=ORIENTED_EDGE('',*,*,#9835,.F.);
#14448=ORIENTED_EDGE('',*,*,#9839,.F.);
#14449=ORIENTED_EDGE('',*,*,#9842,.F.);
#14450=ORIENTED_EDGE('',*,*,#9845,.F.);
#14451=ORIENTED_EDGE('',*,*,#9848,.F.);
#14452=ORIENTED_EDGE('',*,*,#9851,.F.);
#14453=ORIENTED_EDGE('',*,*,#9882,.F.);
#14454=ORIENTED_EDGE('',*,*,#9850,.T.);
#14455=ORIENTED_EDGE('',*,*,#9876,.T.);
#14456=ORIENTED_EDGE('',*,*,#9883,.F.);
#14457=ORIENTED_EDGE('',*,*,#9882,.T.);
#14458=ORIENTED_EDGE('',*,*,#9884,.F.);
#14459=ORIENTED_EDGE('',*,*,#9885,.F.);
#14460=ORIENTED_EDGE('',*,*,#9886,.T.);
#14461=ORIENTED_EDGE('',*,*,#9884,.T.);
#14462=ORIENTED_EDGE('',*,*,#9886,.F.);
#14463=ORIENTED_EDGE('',*,*,#9887,.F.);
#14464=ORIENTED_EDGE('',*,*,#9888,.T.);
#14465=ORIENTED_EDGE('',*,*,#9885,.T.);
#14466=ORIENTED_EDGE('',*,*,#9888,.F.);
#14467=ORIENTED_EDGE('',*,*,#9887,.T.);
#14468=ORIENTED_EDGE('',*,*,#9881,.T.);
#14469=ORIENTED_EDGE('',*,*,#9879,.T.);
#14470=ORIENTED_EDGE('',*,*,#9877,.T.);
#14471=ORIENTED_EDGE('',*,*,#9836,.F.);
#14472=ORIENTED_EDGE('',*,*,#9889,.F.);
#14473=ORIENTED_EDGE('',*,*,#9890,.T.);
#14474=ORIENTED_EDGE('',*,*,#9873,.T.);
#14475=ORIENTED_EDGE('',*,*,#9883,.T.);
#14476=ORIENTED_EDGE('',*,*,#9874,.T.);
#14477=ORIENTED_EDGE('',*,*,#9890,.F.);
#14478=ORIENTED_EDGE('',*,*,#9889,.T.);
#15949=PLANE('',#18656);
#15950=PLANE('',#18663);
#15951=PLANE('',#18669);
#15952=PLANE('',#18672);
#16830=ADVANCED_FACE('',(#3021),#362,.T.);
#16831=ADVANCED_FACE('',(#3022),#363,.T.);
#16832=ADVANCED_FACE('',(#3023),#364,.T.);
#16833=ADVANCED_FACE('',(#3024),#365,.T.);
#16834=ADVANCED_FACE('',(#3025),#366,.T.);
#16835=ADVANCED_FACE('',(#3026),#367,.T.);
#16836=ADVANCED_FACE('',(#3027),#368,.T.);
#16837=ADVANCED_FACE('',(#3028),#369,.T.);
#16838=ADVANCED_FACE('',(#3029),#370,.T.);
#16839=ADVANCED_FACE('',(#3030),#371,.T.);
#16840=ADVANCED_FACE('',(#3031),#372,.T.);
#16841=ADVANCED_FACE('',(#3032),#373,.T.);
#16842=ADVANCED_FACE('',(#3033),#15949,.F.);
#16843=ADVANCED_FACE('',(#3034),#78,.F.);
#16844=ADVANCED_FACE('',(#3035),#374,.T.);
#16845=ADVANCED_FACE('',(#3036),#79,.F.);
#16846=ADVANCED_FACE('',(#3037),#375,.T.);
#16847=ADVANCED_FACE('',(#3038),#15950,.T.);
#16848=ADVANCED_FACE('',(#3039),#1029,.T.);
#16849=ADVANCED_FACE('',(#3040),#376,.T.);
#16850=ADVANCED_FACE('',(#3041,#1465),#15951,.T.);
#16851=ADVANCED_FACE('',(#3042),#1030,.T.);
#16852=ADVANCED_FACE('',(#3043),#15952,.T.);
#17075=CLOSED_SHELL('',(#16830,#16831,#16832,#16833,#16834,#16835,#16836,
#16837,#16838,#16839,#16840,#16841,#16842,#16843,#16844,#16845,#16846,#16847,
#16848,#16849,#16850,#16851,#16852));
#18641=AXIS2_PLACEMENT_3D('',#31897,#22586,#22587);
#18642=AXIS2_PLACEMENT_3D('',#31898,#22588,#22589);
#18643=AXIS2_PLACEMENT_3D('',#31914,#22591,#22592);
#18644=AXIS2_PLACEMENT_3D('',#31922,#22593,#22594);
#18645=AXIS2_PLACEMENT_3D('',#31970,#22596,#22597);
#18646=AXIS2_PLACEMENT_3D('',#32021,#22599,#22600);
#18647=AXIS2_PLACEMENT_3D('',#32072,#22602,#22603);
#18648=AXIS2_PLACEMENT_3D('',#32120,#22605,#22606);
#18649=AXIS2_PLACEMENT_3D('',#32174,#22608,#22609);
#18650=AXIS2_PLACEMENT_3D('',#32186,#22611,#22612);
#18651=AXIS2_PLACEMENT_3D('',#32192,#22613,#22614);
#18652=AXIS2_PLACEMENT_3D('',#32217,#22616,#22617);
#18653=AXIS2_PLACEMENT_3D('',#32242,#22619,#22620);
#18654=AXIS2_PLACEMENT_3D('',#32266,#22622,#22623);
#18655=AXIS2_PLACEMENT_3D('',#32292,#22625,#22626);
#18656=AXIS2_PLACEMENT_3D('',#32316,#22628,#22629);
#18657=AXIS2_PLACEMENT_3D('',#32407,#22630,#22631);
#18658=AXIS2_PLACEMENT_3D('',#32409,#22632,#22633);
#18659=AXIS2_PLACEMENT_3D('',#32800,#22634,#22635);
#18660=AXIS2_PLACEMENT_3D('',#32802,#22636,#22637);
#18661=AXIS2_PLACEMENT_3D('',#33100,#22638,#22639);
#18662=AXIS2_PLACEMENT_3D('',#33101,#22640,#22641);
#18663=AXIS2_PLACEMENT_3D('',#33102,#22642,#22643);
#18664=AXIS2_PLACEMENT_3D('',#33104,#22644,#22645);
#18665=AXIS2_PLACEMENT_3D('',#33105,#22646,#22647);
#18666=AXIS2_PLACEMENT_3D('',#33107,#22648,#22649);
#18667=AXIS2_PLACEMENT_3D('',#33109,#22651,#22652);
#18668=AXIS2_PLACEMENT_3D('',#33111,#22653,#22654);
#18669=AXIS2_PLACEMENT_3D('',#33113,#22656,#22657);
#18670=AXIS2_PLACEMENT_3D('',#33114,#22658,#22659);
#18671=AXIS2_PLACEMENT_3D('',#33116,#22660,#22661);
#18672=AXIS2_PLACEMENT_3D('',#33118,#22663,#22664);
#22586=DIRECTION('axis',(0.,0.,1.));
#22587=DIRECTION('refdir',(1.,0.,0.));
#22588=DIRECTION('center_axis',(1.,0.,0.));
#22589=DIRECTION('ref_axis',(0.,1.,0.));
#22590=DIRECTION('',(-1.,0.,0.));
#22591=DIRECTION('center_axis',(-1.,0.,0.));
#22592=DIRECTION('ref_axis',(0.,1.,0.));
#22593=DIRECTION('center_axis',(1.,0.,0.));
#22594=DIRECTION('ref_axis',(0.,1.,0.));
#22595=DIRECTION('',(-1.,0.,0.));
#22596=DIRECTION('center_axis',(1.,0.,0.));
#22597=DIRECTION('ref_axis',(0.,1.,0.));
#22598=DIRECTION('',(-1.,0.,0.));
#22599=DIRECTION('center_axis',(1.,0.,0.));
#22600=DIRECTION('ref_axis',(0.,1.,0.));
#22601=DIRECTION('',(-1.,0.,0.));
#22602=DIRECTION('center_axis',(1.,0.,0.));
#22603=DIRECTION('ref_axis',(0.,1.,0.));
#22604=DIRECTION('',(-1.,0.,0.));
#22605=DIRECTION('center_axis',(1.,0.,0.));
#22606=DIRECTION('ref_axis',(0.,1.,0.));
#22607=DIRECTION('',(-1.,0.,0.));
#22608=DIRECTION('center_axis',(1.,0.,0.));
#22609=DIRECTION('ref_axis',(0.,-0.289393351880426,-0.957210263154032));
#22610=DIRECTION('',(1.,0.,0.));
#22611=DIRECTION('center_axis',(1.,0.,0.));
#22612=DIRECTION('ref_axis',(0.,1.,9.11763443140316E-15));
#22613=DIRECTION('center_axis',(1.,0.,0.));
#22614=DIRECTION('ref_axis',(0.,1.,9.11763443140316E-15));
#22615=DIRECTION('',(1.,0.,0.));
#22616=DIRECTION('center_axis',(1.,0.,0.));
#22617=DIRECTION('ref_axis',(0.,1.,9.11763443140316E-15));
#22618=DIRECTION('',(1.,0.,0.));
#22619=DIRECTION('center_axis',(1.,0.,0.));
#22620=DIRECTION('ref_axis',(0.,1.,9.11763443140316E-15));
#22621=DIRECTION('',(1.,0.,0.));
#22622=DIRECTION('center_axis',(1.,0.,0.));
#22623=DIRECTION('ref_axis',(0.,1.,9.11763443140316E-15));
#22624=DIRECTION('',(1.,0.,0.));
#22625=DIRECTION('center_axis',(1.,0.,0.));
#22626=DIRECTION('ref_axis',(0.,1.,9.11763443140316E-15));
#22627=DIRECTION('',(1.,0.,0.));
#22628=DIRECTION('center_axis',(1.,0.,0.));
#22629=DIRECTION('ref_axis',(0.,0.,-1.));
#22630=DIRECTION('center_axis',(-1.,0.,0.));
#22631=DIRECTION('ref_axis',(0.,1.,0.));
#22632=DIRECTION('center_axis',(-1.,0.,0.));
#22633=DIRECTION('ref_axis',(0.,1.,0.));
#22634=DIRECTION('center_axis',(1.,0.,0.));
#22635=DIRECTION('ref_axis',(0.,0.889041585325826,0.457826451356126));
#22636=DIRECTION('center_axis',(-1.,0.,0.));
#22637=DIRECTION('ref_axis',(0.,1.,9.11763443140316E-15));
#22638=DIRECTION('center_axis',(1.,0.,0.));
#22639=DIRECTION('ref_axis',(0.,0.929925526089149,-0.367747897244593));
#22640=DIRECTION('center_axis',(-1.,0.,0.));
#22641=DIRECTION('ref_axis',(0.,1.,0.));
#22642=DIRECTION('center_axis',(-1.,0.,0.));
#22643=DIRECTION('ref_axis',(0.,0.,1.));
#22644=DIRECTION('center_axis',(1.,0.,0.));
#22645=DIRECTION('ref_axis',(0.,0.,-1.));
#22646=DIRECTION('center_axis',(1.,0.,0.));
#22647=DIRECTION('ref_axis',(0.,1.,0.));
#22648=DIRECTION('center_axis',(1.,0.,0.));
#22649=DIRECTION('ref_axis',(0.,0.,-1.));
#22650=DIRECTION('',(-0.707106781186547,0.707106781186548,8.65956056235494E-17));
#22651=DIRECTION('center_axis',(1.,0.,0.));
#22652=DIRECTION('ref_axis',(0.,1.,0.));
#22653=DIRECTION('center_axis',(1.,0.,0.));
#22654=DIRECTION('ref_axis',(0.,0.,-1.));
#22655=DIRECTION('',(-1.,0.,0.));
#22656=DIRECTION('center_axis',(1.,0.,0.));
#22657=DIRECTION('ref_axis',(0.,0.,-1.));
#22658=DIRECTION('center_axis',(-1.,0.,0.));
#22659=DIRECTION('ref_axis',(0.,1.,0.));
#22660=DIRECTION('center_axis',(1.,0.,0.));
#22661=DIRECTION('ref_axis',(0.,0.,-1.));
#22662=DIRECTION('',(-0.707106781186544,-0.707106781186551,-8.65956056235498E-17));
#22663=DIRECTION('center_axis',(1.,0.,0.));
#22664=DIRECTION('ref_axis',(0.,0.,-1.));
#31897=CARTESIAN_POINT('',(0.,0.,0.));
#31898=CARTESIAN_POINT('Origin',(25.6,0.,0.));
#31899=CARTESIAN_POINT('',(22.9221761170896,-2.94337932284574,0.0024246877538029));
#31900=CARTESIAN_POINT('',(22.7778238829104,-2.94393084859299,0.00289653660730527));
#31901=CARTESIAN_POINT('',(25.6,-2.942,-3.60291088309151E-16));
#31902=CARTESIAN_POINT('',(22.6,1.28892185405323,2.64462557919718));
#31903=CARTESIAN_POINT('Ctrl Pts',(22.9221761170896,-2.94337932284574,0.0024246877538029));
#31904=CARTESIAN_POINT('Ctrl Pts',(22.912754340928,-2.9448569196983,0.17632691862541));
#31905=CARTESIAN_POINT('Ctrl Pts',(22.9033325647665,-2.93071733453316,0.349980573695374));
#31906=CARTESIAN_POINT('Ctrl Pts',(22.8939107886049,-2.90008429939073,0.520661013315647));
#31907=CARTESIAN_POINT('Ctrl Pts',(22.8419820569707,-2.73124833536721,1.46137734877704));
#31908=CARTESIAN_POINT('Ctrl Pts',(22.7900533253365,-2.06138509115311,2.31177528194959));
#31909=CARTESIAN_POINT('Ctrl Pts',(22.7381245937023,-1.186342977627,2.69686178609481));
#31910=CARTESIAN_POINT('Ctrl Pts',(22.6920830624682,-0.410505064140464,
3.0382907359358));
#31911=CARTESIAN_POINT('Ctrl Pts',(22.6460415312341,0.526626295037523,3.01393307256905));
#31912=CARTESIAN_POINT('Ctrl Pts',(22.6,1.291939685441,2.64724960214527));
#31913=CARTESIAN_POINT('',(22.6,-1.28892185405321,2.64462557919718));
#31914=CARTESIAN_POINT('Origin',(22.6,0.,0.));
#31915=CARTESIAN_POINT('Ctrl Pts',(22.6,-1.28892185405321,2.64462557919718));
#31916=CARTESIAN_POINT('Ctrl Pts',(22.6519287316342,-2.15180458522763,2.22407893605632));
#31917=CARTESIAN_POINT('Ctrl Pts',(22.7038574632684,-2.78633791211509,1.35244859465509));
#31918=CARTESIAN_POINT('Ctrl Pts',(22.7557861949026,-2.91785469712274,0.407185074986569));
#31919=CARTESIAN_POINT('Ctrl Pts',(22.7631320909052,-2.93645920747492,0.273467048529401));
#31920=CARTESIAN_POINT('Ctrl Pts',(22.7704779869078,-2.94499773028714,0.138275530460612));
#31921=CARTESIAN_POINT('Ctrl Pts',(22.7778238829104,-2.94393084859299,0.00289653660730527));
#31922=CARTESIAN_POINT('Origin',(25.6,0.,0.));
#31923=CARTESIAN_POINT('',(23.9221761170896,-2.9383190595815,-0.00138042702469643));
#31924=CARTESIAN_POINT('',(23.7778238829104,-2.93785684534219,-0.000854546637487877));
#31925=CARTESIAN_POINT('',(25.6,-2.942,-3.60291088309151E-16));
#31926=CARTESIAN_POINT('Ctrl Pts',(23.9221761170896,-2.9383190595815,-0.00138042702469643));
#31927=CARTESIAN_POINT('Ctrl Pts',(23.8909933973998,-2.93576543917648,0.576735544293962));
#31928=CARTESIAN_POINT('Ctrl Pts',(23.8598106777101,-2.77025503775714,1.15620073583879));
#31929=CARTESIAN_POINT('Ctrl Pts',(23.8286279580203,-2.45196769155219,1.63386091512667));
#31930=CARTESIAN_POINT('Ctrl Pts',(23.7766992263861,-1.92192225779668,2.42931068696698));
#31931=CARTESIAN_POINT('Ctrl Pts',(23.7247704947519,-0.968189696573736,
2.94243073120691));
#31932=CARTESIAN_POINT('Ctrl Pts',(23.6728417631178,-0.0123243431917003,
2.94643266533865));
#31933=CARTESIAN_POINT('Ctrl Pts',(23.6209130314836,0.943541010190328,2.95043459947038));
#31934=CARTESIAN_POINT('Ctrl Pts',(23.5689842998494,1.90153915573145,2.44531842349393));
#31935=CARTESIAN_POINT('Ctrl Pts',(23.5170555682152,2.43821811361518,1.65431992343549));
#31936=CARTESIAN_POINT('Ctrl Pts',(23.465126836581,2.97489707149892,0.863321423377055));
#31937=CARTESIAN_POINT('Ctrl Pts',(23.4131981049468,3.09025684172528,-0.213559400763362));
#31938=CARTESIAN_POINT('Ctrl Pts',(23.3612693733126,2.73332327778208,-1.10027216939385));
#31939=CARTESIAN_POINT('Ctrl Pts',(23.3093406416784,2.37638971383888,-1.98698493802435));
#31940=CARTESIAN_POINT('Ctrl Pts',(23.2574119100442,1.54716281572612,-2.68352965114492));
#31941=CARTESIAN_POINT('Ctrl Pts',(23.20548317841,0.612137108554167,-2.88214374660199));
#31942=CARTESIAN_POINT('Ctrl Pts',(23.1535544467758,-0.322888598617789,
-3.08075784205906));
#31943=CARTESIAN_POINT('Ctrl Pts',(23.1016257151416,-1.36371311484895,-2.78144131985263));
#31944=CARTESIAN_POINT('Ctrl Pts',(23.0496969835075,-2.05022103104806,-2.1162656898743));
#31945=CARTESIAN_POINT('Ctrl Pts',(23.0071900280348,-2.61217123678476,-1.57177731137621));
#31946=CARTESIAN_POINT('Ctrl Pts',(22.9646830725622,-2.93671304861665,-0.782146528701403));
#31947=CARTESIAN_POINT('Ctrl Pts',(22.9221761170896,-2.94337932284574,0.0024246877538029));
#31948=CARTESIAN_POINT('Ctrl Pts',(22.7778238829104,-2.94393084859299,0.00289653660730527));
#31949=CARTESIAN_POINT('Ctrl Pts',(22.822406718542,-2.93745585749709,-0.818729501766297));
#31950=CARTESIAN_POINT('Ctrl Pts',(22.8669895541736,-2.57717788935255,-1.64726097453814));
#31951=CARTESIAN_POINT('Ctrl Pts',(22.9115723898051,-1.96605887355123,-2.19521297425806));
#31952=CARTESIAN_POINT('Ctrl Pts',(22.9635011214393,-1.25424602184426,-2.83345080589834));
#31953=CARTESIAN_POINT('Ctrl Pts',(23.0154298530735,-0.202120075302478,
-3.09102977124308));
#31954=CARTESIAN_POINT('Ctrl Pts',(23.0673585847077,0.724516079376799,-2.85579333374966));
#31955=CARTESIAN_POINT('Ctrl Pts',(23.1192873163419,1.65115223405607,-2.62055689625624));
#31956=CARTESIAN_POINT('Ctrl Pts',(23.1712160479761,2.45229859687285,-1.89250505592465));
#31957=CARTESIAN_POINT('Ctrl Pts',(23.2231447796103,2.77422274277707,-0.992606024168016));
#31958=CARTESIAN_POINT('Ctrl Pts',(23.2750735112445,3.09614688868129,-0.0927069924113744));
#31959=CARTESIAN_POINT('Ctrl Pts',(23.3270022428787,2.93884881767296,0.979039230770322));
#31960=CARTESIAN_POINT('Ctrl Pts',(23.3789309745129,2.3716618413383,1.74848753980998));
#31961=CARTESIAN_POINT('Ctrl Pts',(23.430859706147,1.80447486500363,2.51793584884963));
#31962=CARTESIAN_POINT('Ctrl Pts',(23.4827884377812,0.827398983342636,2.98508624374724));
#31963=CARTESIAN_POINT('Ctrl Pts',(23.5347171694154,-0.127590825323999,
2.94366917333447));
#31964=CARTESIAN_POINT('Ctrl Pts',(23.5866459010496,-1.08258063399063,2.9022521029217));
#31965=CARTESIAN_POINT('Ctrl Pts',(23.6385746326838,-2.01548436966291,2.35226756719854));
#31966=CARTESIAN_POINT('Ctrl Pts',(23.690503364318,-2.5140002246829,1.53670433537425));
#31967=CARTESIAN_POINT('Ctrl Pts',(23.7196102038488,-2.79342590174055,1.07956880810663));
#31968=CARTESIAN_POINT('Ctrl Pts',(23.7487170433796,-2.93637680815486,0.538994508137228));
#31969=CARTESIAN_POINT('Ctrl Pts',(23.7778238829104,-2.93785684534219,-0.000854546637487877));
#31970=CARTESIAN_POINT('Origin',(25.6,0.,0.));
#31971=CARTESIAN_POINT('',(24.9221761170896,-2.94641400997859,0.000320893440124217));
#31972=CARTESIAN_POINT('',(24.7778238829104,-2.94641005469739,-0.000335482700479716));
#31973=CARTESIAN_POINT('',(25.6,-2.942,-3.60291088309151E-16));
#31974=CARTESIAN_POINT('Ctrl Pts',(24.9221761170896,-2.94641400997859,0.000320893440124217));
#31975=CARTESIAN_POINT('Ctrl Pts',(24.9211611855058,-2.94644390539513,0.0190039752988624));
#31976=CARTESIAN_POINT('Ctrl Pts',(24.9201462539221,-2.94628096860413,0.0376865226429225));
#31977=CARTESIAN_POINT('Ctrl Pts',(24.9191313223383,-2.94592358009294,0.0563653494972846));
#31978=CARTESIAN_POINT('Ctrl Pts',(24.8672025907041,-2.92763788243231,1.01206305610313));
#31979=CARTESIAN_POINT('Ctrl Pts',(24.8152738590699,-2.4003101053229,1.9580211429691));
#31980=CARTESIAN_POINT('Ctrl Pts',(24.7633451274357,-1.59702395175339,2.47611740807419));
#31981=CARTESIAN_POINT('Ctrl Pts',(24.7114163958015,-0.793737798183883,
2.99421367317928));
#31982=CARTESIAN_POINT('Ctrl Pts',(24.6594876641674,0.285506731845734,3.08444811652349));
#31983=CARTESIAN_POINT('Ctrl Pts',(24.6075589325332,1.16367382457068,2.70693656051822));
#31984=CARTESIAN_POINT('Ctrl Pts',(24.555630200899,2.04184091729562,2.32942500451294));
#31985=CARTESIAN_POINT('Ctrl Pts',(24.5037014692648,2.7189305727159,1.48416744915818));
#31986=CARTESIAN_POINT('Ctrl Pts',(24.4517727376306,2.8956628730315,0.544774888775652));
#31987=CARTESIAN_POINT('Ctrl Pts',(24.3998440059964,3.07239517334711,-0.394617671606881));
#31988=CARTESIAN_POINT('Ctrl Pts',(24.3479152743622,2.74877011855805,-1.42814523701718));
#31989=CARTESIAN_POINT('Ctrl Pts',(24.295986542728,2.06783319808421,-2.09897820914092));
#31990=CARTESIAN_POINT('Ctrl Pts',(24.2440578110938,1.38689627761036,-2.76981118126465));
#31991=CARTESIAN_POINT('Ctrl Pts',(24.1921290794596,0.348647491451722,-3.07794956010182));
#31992=CARTESIAN_POINT('Ctrl Pts',(24.1402003478254,-0.587998308823754,
-2.8871954022964));
#31993=CARTESIAN_POINT('Ctrl Pts',(24.0882716161913,-1.52464410909923,-2.69644124449098));
#31994=CARTESIAN_POINT('Ctrl Pts',(24.0363428845571,-2.35968692349154,-2.00679455004298));
#31995=CARTESIAN_POINT('Ctrl Pts',(23.9844141529229,-2.72402917754366,-1.12308145309864));
#31996=CARTESIAN_POINT('Ctrl Pts',(23.9636681409785,-2.86958730146767,-0.770029840095521));
#31997=CARTESIAN_POINT('Ctrl Pts',(23.942922129034,-2.94001799540079,-0.386003736523308));
#31998=CARTESIAN_POINT('Ctrl Pts',(23.9221761170896,-2.9383190595815,-0.00138042702469643));
#31999=CARTESIAN_POINT('Ctrl Pts',(23.7778238829104,-2.93785684534219,-0.000854546637487877));
#32000=CARTESIAN_POINT('Ctrl Pts',(23.8006457750138,-2.9390173027997,-0.42413570937398));
#32001=CARTESIAN_POINT('Ctrl Pts',(23.8234676671172,-2.85320560862381,-0.846971012582013));
#32002=CARTESIAN_POINT('Ctrl Pts',(23.8462895592206,-2.67801351714517,-1.22879127448483));
#32003=CARTESIAN_POINT('Ctrl Pts',(23.8982182908548,-2.27938298021973,-2.09758172459419));
#32004=CARTESIAN_POINT('Ctrl Pts',(23.950147022489,-1.41799393200115,-2.75402069688747));
#32005=CARTESIAN_POINT('Ctrl Pts',(24.0020757541231,-0.474601113597208,
-2.90798448590835));
#32006=CARTESIAN_POINT('Ctrl Pts',(24.0540044857573,0.468791704806728,-3.06194827492923));
#32007=CARTESIAN_POINT('Ctrl Pts',(24.1059332173915,1.49418829339602,-2.71343688067772));
#32008=CARTESIAN_POINT('Ctrl Pts',(24.1578619490257,2.14836063534518,-2.0164811236668));
#32009=CARTESIAN_POINT('Ctrl Pts',(24.2097906806599,2.80253297729433,-1.31952536665587));
#32010=CARTESIAN_POINT('Ctrl Pts',(24.2617194122941,3.08548107260335,-0.274125246885542));
#32011=CARTESIAN_POINT('Ctrl Pts',(24.3136481439283,2.87213594284245,0.657635574862683));
#32012=CARTESIAN_POINT('Ctrl Pts',(24.3655768755625,2.65879081308155,1.58939639661091));
#32013=CARTESIAN_POINT('Ctrl Pts',(24.4175056071966,1.94915245825073,2.40751792033702));
#32014=CARTESIAN_POINT('Ctrl Pts',(24.4694343388308,1.05688918030864,2.75038672001481));
#32015=CARTESIAN_POINT('Ctrl Pts',(24.521363070465,0.164625902366541,3.0932555196926));
#32016=CARTESIAN_POINT('Ctrl Pts',(24.5732918020992,-0.910262298686838,
2.96087159532206));
#32017=CARTESIAN_POINT('Ctrl Pts',(24.6252205337334,-1.69266594113809,2.41174795315879));
#32018=CARTESIAN_POINT('Ctrl Pts',(24.6760883167924,-2.45908440537369,1.87384337850255));
#32019=CARTESIAN_POINT('Ctrl Pts',(24.7269560998514,-2.94484764344756,0.936053831091904));
#32020=CARTESIAN_POINT('Ctrl Pts',(24.7778238829104,-2.94641005469739,-0.000335482700479716));
#32021=CARTESIAN_POINT('Origin',(25.6,0.,0.));
#32022=CARTESIAN_POINT('',(25.9221761170896,-2.93786869100257,0.000876386695073395));
#32023=CARTESIAN_POINT('',(25.7778238829104,-2.93833233985647,0.00139222834412371));
#32024=CARTESIAN_POINT('',(25.6,-2.942,-3.60291088309151E-16));
#32025=CARTESIAN_POINT('Ctrl Pts',(25.9221761170896,-2.93786869100257,0.000876386695073395));
#32026=CARTESIAN_POINT('Ctrl Pts',(25.8994002419776,-2.93904020397999,0.423294701449549));
#32027=CARTESIAN_POINT('Ctrl Pts',(25.8766243668657,-2.85358407529444,0.845261266561695));
#32028=CARTESIAN_POINT('Ctrl Pts',(25.8538484917537,-2.67907431130908,1.22645975976682));
#32029=CARTESIAN_POINT('Ctrl Pts',(25.8019197601195,-2.28119406929874,2.09558791206413));
#32030=CARTESIAN_POINT('Ctrl Pts',(25.7499910284854,-1.42038210979013,2.75278947109579));
#32031=CARTESIAN_POINT('Ctrl Pts',(25.6980622968512,-0.477125112358299,
2.90757535073352));
#32032=CARTESIAN_POINT('Ctrl Pts',(25.646133565217,0.466131885073529,3.06236123037125));
#32033=CARTESIAN_POINT('Ctrl Pts',(25.5942048335828,1.49183392042857,2.71473143061506));
#32034=CARTESIAN_POINT('Ctrl Pts',(25.5422761019486,2.14661136587812,2.01834149796711));
#32035=CARTESIAN_POINT('Ctrl Pts',(25.4903473703144,2.80138881132767,1.32195156531916));
#32036=CARTESIAN_POINT('Ctrl Pts',(25.4384186386802,3.08524166687174,0.276801499779447));
#32037=CARTESIAN_POINT('Ctrl Pts',(25.386489907046,2.87270439640652,-0.655142892352426));
#32038=CARTESIAN_POINT('Ctrl Pts',(25.3345611754118,2.6601671259413,-1.5870872844843));
#32039=CARTESIAN_POINT('Ctrl Pts',(25.2826324437776,1.95123972946679,-2.40582600320835));
#32040=CARTESIAN_POINT('Ctrl Pts',(25.2307037121434,1.05927455670128,-2.74946907721497));
#32041=CARTESIAN_POINT('Ctrl Pts',(25.1787749805093,0.16730938393577,-3.0931121512216));
#32042=CARTESIAN_POINT('Ctrl Pts',(25.1268462488751,-0.907693565120746,
-2.9616595805108));
#32043=CARTESIAN_POINT('Ctrl Pts',(25.0749175172409,-1.69057323054308,-2.41321463198254));
#32044=CARTESIAN_POINT('Ctrl Pts',(25.0240037171904,-2.45815174622199,-1.87548887652329));
#32045=CARTESIAN_POINT('Ctrl Pts',(24.97308991714,-2.94491431356086,-0.936911437587762));
#32046=CARTESIAN_POINT('Ctrl Pts',(24.9221761170896,-2.94641400997859,0.000320893440124217));
#32047=CARTESIAN_POINT('Ctrl Pts',(24.7778238829104,-2.94641005469739,-0.000335482700479716));
#32048=CARTESIAN_POINT('Ctrl Pts',(24.7788848314856,-2.94644264188499,-0.0198657403321496));
#32049=CARTESIAN_POINT('Ctrl Pts',(24.7799457800608,-2.94626459502485,-0.0393953888428549));
#32050=CARTESIAN_POINT('Ctrl Pts',(24.781006728636,-2.94587406733219,-0.0589207873412386));
#32051=CARTESIAN_POINT('Ctrl Pts',(24.8329354602702,-2.92675946722594,-1.01460252572203));
#32052=CARTESIAN_POINT('Ctrl Pts',(24.8848641919044,-2.3986111831643,-1.96010264252762));
#32053=CARTESIAN_POINT('Ctrl Pts',(24.9367929235386,-1.59487577768028,-2.47750198725934));
#32054=CARTESIAN_POINT('Ctrl Pts',(24.9887216551728,-0.791140372196265,
-2.99490133199106));
#32055=CARTESIAN_POINT('Ctrl Pts',(25.0406503868069,0.288182154710141,-3.08419990464891));
#32056=CARTESIAN_POINT('Ctrl Pts',(25.0925791184411,1.16602155650292,-2.70592667620281));
#32057=CARTESIAN_POINT('Ctrl Pts',(25.1445078500753,2.0438609582957,-2.32765344775672));
#32058=CARTESIAN_POINT('Ctrl Pts',(25.1964365817095,2.72021723497484,-1.48180841820668));
#32059=CARTESIAN_POINT('Ctrl Pts',(25.2483653133437,2.89613471145009,-0.54226290020962));
#32060=CARTESIAN_POINT('Ctrl Pts',(25.3002940449779,3.07205218792534,0.39728261778744));
#32061=CARTESIAN_POINT('Ctrl Pts',(25.3522227766121,2.74753086419669,1.43052862423153));
#32062=CARTESIAN_POINT('Ctrl Pts',(25.4041515082463,2.06601214166399,2.1007710646963));
#32063=CARTESIAN_POINT('Ctrl Pts',(25.4560802398804,1.38449341913129,2.77101350516106));
#32064=CARTESIAN_POINT('Ctrl Pts',(25.5080089715146,0.345977297794549,3.07825237964651));
#32065=CARTESIAN_POINT('Ctrl Pts',(25.5599377031488,-0.590502677571841,
2.8866852803957));
#32066=CARTESIAN_POINT('Ctrl Pts',(25.611866434783,-1.52698265293823,2.69511818114489));
#32067=CARTESIAN_POINT('Ctrl Pts',(25.6637951664172,-2.36142648233428,2.00474510815782));
#32068=CARTESIAN_POINT('Ctrl Pts',(25.7157238980514,-2.72500240918793,1.12071725070303));
#32069=CARTESIAN_POINT('Ctrl Pts',(25.7364238930044,-2.86993219302934,0.768323275118707));
#32070=CARTESIAN_POINT('Ctrl Pts',(25.7571238879574,-2.94004086870962,0.38515747266671));
#32071=CARTESIAN_POINT('Ctrl Pts',(25.7778238829104,-2.93833233985647,0.00139222834412371));
#32072=CARTESIAN_POINT('Origin',(25.6,0.,0.));
#32073=CARTESIAN_POINT('',(26.9221761170896,-2.94442477429212,-0.00197218427072376));
#32074=CARTESIAN_POINT('',(26.7778238829104,-2.94339904745569,-0.00227025699168395));
#32075=CARTESIAN_POINT('',(25.6,-2.942,-3.60291088309151E-16));
#32076=CARTESIAN_POINT('Ctrl Pts',(26.9221761170896,-2.94442477429212,-0.00197218427072376));
#32077=CARTESIAN_POINT('Ctrl Pts',(26.8776392984494,-2.93802580261633,0.819340609163623));
#32078=CARTESIAN_POINT('Ctrl Pts',(26.8331024798093,-2.57794208161663,1.6455819227055));
#32079=CARTESIAN_POINT('Ctrl Pts',(26.7885656611692,-1.96775235997052,2.19307773506812));
#32080=CARTESIAN_POINT('Ctrl Pts',(26.736636929535,-1.25628757041458,2.831443114076));
#32081=CARTESIAN_POINT('Ctrl Pts',(26.6847081979008,-0.204805367471877,
3.09085587275804));
#32082=CARTESIAN_POINT('Ctrl Pts',(26.6327794662666,0.721931053663677,2.85665174834169));
#32083=CARTESIAN_POINT('Ctrl Pts',(26.5808507346324,1.64866747479923,2.62244762392534));
#32084=CARTESIAN_POINT('Ctrl Pts',(26.5289220029982,2.45065811412763,1.89462661641059));
#32085=CARTESIAN_POINT('Ctrl Pts',(26.476993271364,2.77341506728714,0.99489296823238));
#32086=CARTESIAN_POINT('Ctrl Pts',(26.4250645397298,3.09617202044665,0.0951593200541696));
#32087=CARTESIAN_POINT('Ctrl Pts',(26.3731358080956,2.93969528743728,-0.976486968787502));
#32088=CARTESIAN_POINT('Ctrl Pts',(26.3212070764614,2.37314939075441,-1.7463688848073));
#32089=CARTESIAN_POINT('Ctrl Pts',(26.2692783448273,1.80660349407155,-2.5162508008271));
#32090=CARTESIAN_POINT('Ctrl Pts',(26.2173496131931,0.829988433715184,-2.98436834402501));
#32091=CARTESIAN_POINT('Ctrl Pts',(26.1654208815589,-0.125023259080066,
-2.94380911502955));
#32092=CARTESIAN_POINT('Ctrl Pts',(26.1134921499247,-1.08003495187532,-2.90324988603409));
#32093=CARTESIAN_POINT('Ctrl Pts',(26.0615634182905,-2.01344327710945,-2.35401388484526));
#32094=CARTESIAN_POINT('Ctrl Pts',(26.0096346866563,-2.51267317747048,-1.53886851146936));
#32095=CARTESIAN_POINT('Ctrl Pts',(25.9804818301341,-2.79294148364365,-1.08124485368015));
#32096=CARTESIAN_POINT('Ctrl Pts',(25.9513289736118,-2.93636916795125,-0.539814166878388));
#32097=CARTESIAN_POINT('Ctrl Pts',(25.9221761170896,-2.93786869100257,0.000876386695073395));
#32098=CARTESIAN_POINT('Ctrl Pts',(25.7778238829104,-2.93833233985647,0.00139222834412371));
#32099=CARTESIAN_POINT('Ctrl Pts',(25.8090526195916,-2.93575479344698,-0.577569447229037));
#32100=CARTESIAN_POINT('Ctrl Pts',(25.8402813562728,-2.76972275937453,-1.15789544023111));
#32101=CARTESIAN_POINT('Ctrl Pts',(25.871510092954,-2.45055050830498,-1.6359851748563));
#32102=CARTESIAN_POINT('Ctrl Pts',(25.9234388245882,-1.91981465625711,-2.43097710103833));
#32103=CARTESIAN_POINT('Ctrl Pts',(25.9753675562224,-0.965634927850109,
-2.9432783114799));
#32104=CARTESIAN_POINT('Ctrl Pts',(26.0272962878566,-0.00976743849944818,
-2.94644699891546));
#32105=CARTESIAN_POINT('Ctrl Pts',(26.0792250194907,0.946100050851219,-2.94961568635102));
#32106=CARTESIAN_POINT('Ctrl Pts',(26.1311537511249,1.90365530114555,-2.44365185078057));
#32107=CARTESIAN_POINT('Ctrl Pts',(26.1830824827591,2.43965021452719,-1.65219613439981));
#32108=CARTESIAN_POINT('Ctrl Pts',(26.2350112143933,2.97564512790882,-0.860740418019046));
#32109=CARTESIAN_POINT('Ctrl Pts',(26.2869399460275,3.09007970437777,0.216207179172027));
#32110=CARTESIAN_POINT('Ctrl Pts',(26.3388686776617,2.73237278071044,1.10262609575619));
#32111=CARTESIAN_POINT('Ctrl Pts',(26.3907974092959,2.37466585704312,1.98904501234035));
#32112=CARTESIAN_POINT('Ctrl Pts',(26.4427261409301,1.54481743323954,2.6849352483176));
#32113=CARTESIAN_POINT('Ctrl Pts',(26.4946548725643,0.609628131457622,2.88270688564602));
#32114=CARTESIAN_POINT('Ctrl Pts',(26.5465836041984,-0.325561170324308,
3.08047852297444));
#32115=CARTESIAN_POINT('Ctrl Pts',(26.5985123358326,-1.36609135008459,2.780131561654));
#32116=CARTESIAN_POINT('Ctrl Pts',(26.6504410674668,-2.05203877789913,2.11442230812662));
#32117=CARTESIAN_POINT('Ctrl Pts',(26.692902005948,-2.61292233151529,1.57008704764869));
#32118=CARTESIAN_POINT('Ctrl Pts',(26.7353629444292,-2.93673328995051,0.78147203492828));
#32119=CARTESIAN_POINT('Ctrl Pts',(26.7778238829104,-2.94339904745569,-0.00227025699168395));
#32120=CARTESIAN_POINT('Origin',(25.6,0.,0.));
#32121=CARTESIAN_POINT('',(27.9221761170896,-2.94084529159276,0.00236346891266642));
#32122=CARTESIAN_POINT('',(27.7778238829104,-2.9419205159921,0.00243417433800859));
#32123=CARTESIAN_POINT('',(25.6,-2.942,-3.60291088309151E-16));
#32124=CARTESIAN_POINT('Ctrl Pts',(27.9221761170896,-2.94084529159276,0.00236346891266642));
#32125=CARTESIAN_POINT('Ctrl Pts',(27.9078070865555,-2.94302846982566,0.268201177356569));
#32126=CARTESIAN_POINT('Ctrl Pts',(27.8934380560213,-2.90984722496843,0.533507849845637));
#32127=CARTESIAN_POINT('Ctrl Pts',(27.8790690254872,-2.83909368778622,0.788374135968067));
#32128=CARTESIAN_POINT('Ctrl Pts',(27.827140293853,-2.5833950562207,1.70944413739935));
#32129=CARTESIAN_POINT('Ctrl Pts',(27.7752115622188,-1.83698271972066,2.49415725566241));
#32130=CARTESIAN_POINT('Ctrl Pts',(27.7232828305846,-0.929946677882633,
2.79582967865374));
#32131=CARTESIAN_POINT('Ctrl Pts',(27.6713540989504,-0.0229106360446091,
3.09750210164506));
#32132=CARTESIAN_POINT('Ctrl Pts',(27.6194253673162,1.0447491111314,2.91613382936466));
#32133=CARTESIAN_POINT('Ctrl Pts',(27.567496635682,1.80120320149326,2.33180659887102));
#32134=CARTESIAN_POINT('Ctrl Pts',(27.5155679040478,2.55765729185511,1.74747936837739));
#32135=CARTESIAN_POINT('Ctrl Pts',(27.4636391724136,3.00290572540282,0.760193179670536));
#32136=CARTESIAN_POINT('Ctrl Pts',(27.4117104407794,2.94010093297105,-0.193619427174991));
#32137=CARTESIAN_POINT('Ctrl Pts',(27.3597817091452,2.87729614053928,-1.14743203402053));
#32138=CARTESIAN_POINT('Ctrl Pts',(27.3078529775111,2.30643812212801,-2.06777105900474));
#32139=CARTESIAN_POINT('Ctrl Pts',(27.2559242458769,1.47987354517457,-2.54786020635006));
#32140=CARTESIAN_POINT('Ctrl Pts',(27.2039955142427,0.653308968221138,-3.02794935369537));
#32141=CARTESIAN_POINT('Ctrl Pts',(27.1520667826085,-0.428962167274455,
-3.0677886234018));
#32142=CARTESIAN_POINT('Ctrl Pts',(27.1001380509743,-1.28857750153804,-2.64975754983817));
#32143=CARTESIAN_POINT('Ctrl Pts',(27.0482093193401,-2.14819283580162,-2.23172647627454));
#32144=CARTESIAN_POINT('Ctrl Pts',(26.9962805877059,-2.7851523688332,-1.35582505944085));
#32145=CARTESIAN_POINT('Ctrl Pts',(26.9443518560717,-2.91790844726441,-0.409215351357154));
#32146=CARTESIAN_POINT('Ctrl Pts',(26.9369599430777,-2.93680591212272,-0.274468047094759));
#32147=CARTESIAN_POINT('Ctrl Pts',(26.9295680300836,-2.94548683133442,-0.138287998810961));
#32148=CARTESIAN_POINT('Ctrl Pts',(26.9221761170896,-2.94442477429212,-0.00197218427072376));
#32149=CARTESIAN_POINT('Ctrl Pts',(26.7778238829104,-2.94339904745569,-0.00227025699168395));
#32150=CARTESIAN_POINT('Ctrl Pts',(26.7872916760634,-2.94488535500151,-0.177026401593688));
#32151=CARTESIAN_POINT('Ctrl Pts',(26.7967594692164,-2.93060366699902,-0.351540281644112));
#32152=CARTESIAN_POINT('Ctrl Pts',(26.8062272623694,-2.89966629313921,-0.523049776019018));
#32153=CARTESIAN_POINT('Ctrl Pts',(26.8581559940036,-2.72998170469592,-1.46374106090295));
#32154=CARTESIAN_POINT('Ctrl Pts',(26.9100847256378,-2.05924785194055,-2.31405208493648));
#32155=CARTESIAN_POINT('Ctrl Pts',(26.962013457272,-1.18393581131734,-2.69813679648287));
#32156=CARTESIAN_POINT('Ctrl Pts',(27.0139421889062,-0.308623770694144,
-3.08222150802926));
#32157=CARTESIAN_POINT('Ctrl Pts',(27.0658709205403,0.77126645779688,-3.00007990708851));
#32158=CARTESIAN_POINT('Ctrl Pts',(27.1177996521745,1.57841480666123,-2.48802101020065));
#32159=CARTESIAN_POINT('Ctrl Pts',(27.1697283838087,2.38556315552559,-1.9759621133128));
#32160=CARTESIAN_POINT('Ctrl Pts',(27.2216571154429,2.91996962476327,-1.03398592047784));
#32161=CARTESIAN_POINT('Ctrl Pts',(27.2735858470771,2.9454192977785,-0.0784511552908093));
#32162=CARTESIAN_POINT('Ctrl Pts',(27.3255145787113,2.97086897079373,0.87708360989624));
#32163=CARTESIAN_POINT('Ctrl Pts',(27.3774433103455,2.48736184758648,1.84617694743536));
#32164=CARTESIAN_POINT('Ctrl Pts',(27.4293720419797,1.7086171945732,2.40047429147118));
#32165=CARTESIAN_POINT('Ctrl Pts',(27.4813007736139,0.929872541559935,2.95477163550698));
#32166=CARTESIAN_POINT('Ctrl Pts',(27.5332295052481,-0.144109641259354,
3.09427298603949));
#32167=CARTESIAN_POINT('Ctrl Pts',(27.5851582368823,-1.03862876920953,2.75733027892591));
#32168=CARTESIAN_POINT('Ctrl Pts',(27.6370869685165,-1.93314789715972,2.42038757181232));
#32169=CARTESIAN_POINT('Ctrl Pts',(27.6890157001506,-2.6482039702408,1.60700080705263));
#32170=CARTESIAN_POINT('Ctrl Pts',(27.7409444317848,-2.86771742957133,0.676669149876849));
#32171=CARTESIAN_POINT('Ctrl Pts',(27.75323758216,-2.91968311176705,0.456430630649596));
#32172=CARTESIAN_POINT('Ctrl Pts',(27.7655307325352,-2.94387776538163,0.229638326017039));
#32173=CARTESIAN_POINT('Ctrl Pts',(27.7778238829104,-2.9419205159921,0.00243417433800859));
#32174=CARTESIAN_POINT('Origin',(20.751410108095,0.,0.));
#32175=CARTESIAN_POINT('',(28.251410108095,-2.37081910956327,0.00190535601414123));
#32176=CARTESIAN_POINT('',(28.448589891905,-2.36902607076732,-0.00230475997383739));
#32177=CARTESIAN_POINT('',(20.751410108095,-2.37175,-2.19152050672682E-14));
#32178=CARTESIAN_POINT('',(28.658,1.97801633036407,-1.31405326343373));
#32179=CARTESIAN_POINT('Ctrl Pts',(28.251410108095,-2.37081910956327,0.00190535601414134));
#32180=CARTESIAN_POINT('Ctrl Pts',(28.288969809195,-2.36621855598052,-0.558287395810164));
#32181=CARTESIAN_POINT('Ctrl Pts',(28.3784582419293,-1.89114103981992,-1.89995231291283));
#32182=CARTESIAN_POINT('Ctrl Pts',(28.5139882058976,0.229773146349892,-2.73041805462421));
#32183=CARTESIAN_POINT('Ctrl Pts',(28.6119584687659,1.59534824541231,-1.88115502388143));
#32184=CARTESIAN_POINT('Ctrl Pts',(28.658,1.97801633036407,-1.31405326343373));
#32185=CARTESIAN_POINT('',(28.658,-0.598340649004819,-2.29503519150546));
#32186=CARTESIAN_POINT('Origin',(28.658,0.,0.));
#32187=CARTESIAN_POINT('Ctrl Pts',(28.448589891905,-2.36902607076732,-0.00230475997383763));
#32188=CARTESIAN_POINT('Ctrl Pts',(28.4664645296358,-2.37066543904879,-0.26930526887278));
#32189=CARTESIAN_POINT('Ctrl Pts',(28.5362678990008,-2.20751399255987,-1.30936831204417));
#32190=CARTESIAN_POINT('Ctrl Pts',(28.6060712683658,-1.34715978233134,-2.09980989479535));
#32191=CARTESIAN_POINT('Ctrl Pts',(28.658,-0.598340649004787,-2.29503519150547));
#32192=CARTESIAN_POINT('Origin',(20.751410108095,0.,0.));
#32193=CARTESIAN_POINT('',(27.251410108095,-2.3737047785273,-0.00158991435897493));
#32194=CARTESIAN_POINT('',(27.448589891905,-2.37168592243517,0.00196235655545912));
#32195=CARTESIAN_POINT('',(20.751410108095,-2.37175,-2.19152050672682E-14));
#32196=CARTESIAN_POINT('Ctrl Pts',(27.251410108095,-2.3737047785273,-0.00158991435897499));
#32197=CARTESIAN_POINT('Ctrl Pts',(27.258802021089,-2.37456097628056,-0.111483535411255));
#32198=CARTESIAN_POINT('Ctrl Pts',(27.3181226657173,-2.31839918246699,-0.992509565802802));
#32199=CARTESIAN_POINT('Ctrl Pts',(27.4293720419797,-1.21830985242857,-2.50527411810993));
#32200=CARTESIAN_POINT('Ctrl Pts',(27.5851582368822,1.39917134975873,-2.40892253286906));
#32201=CARTESIAN_POINT('Ctrl Pts',(27.7409444317848,2.77979593014647,-0.183075405908203));
#32202=CARTESIAN_POINT('Ctrl Pts',(27.8967306266874,1.70295911274323,2.20468395989619));
#32203=CARTESIAN_POINT('Ctrl Pts',(28.05251682159,-0.879184332564077,2.64332454430922));
#32204=CARTESIAN_POINT('Ctrl Pts',(28.1707433153925,-2.24915776353418,1.20305343625789));
#32205=CARTESIAN_POINT('Ctrl Pts',(28.2370410775608,-2.37257912077125,0.216215548060989));
#32206=CARTESIAN_POINT('Ctrl Pts',(28.251410108095,-2.37081910956327,0.00190535601414134));
#32207=CARTESIAN_POINT('Ctrl Pts',(27.448589891905,-2.37168592243517,0.00196235655545921));
#32208=CARTESIAN_POINT('Ctrl Pts',(27.488225473164,-2.36659853931644,-0.588598341501691));
#32209=CARTESIAN_POINT('Ctrl Pts',(27.5797897860572,-1.84853809447402,-1.9608582117688));
#32210=CARTESIAN_POINT('Ctrl Pts',(27.7232828305846,0.430422244683163,-2.75224826615359));
#32211=CARTESIAN_POINT('Ctrl Pts',(27.8790690254871,2.52434834774427,-1.17871200290743));
#32212=CARTESIAN_POINT('Ctrl Pts',(28.0348552203897,2.38625876548845,1.43744121743837));
#32213=CARTESIAN_POINT('Ctrl Pts',(28.1906414152923,0.139550436043699,2.78166084946855));
#32214=CARTESIAN_POINT('Ctrl Pts',(28.328552972464,-1.96011683010446,1.79687640253636));
#32215=CARTESIAN_POINT('Ctrl Pts',(28.4145357980016,-2.36590280739046,0.506374662749581));
#32216=CARTESIAN_POINT('Ctrl Pts',(28.448589891905,-2.36902607076732,-0.00230475997383763));
#32217=CARTESIAN_POINT('Origin',(20.751410108095,0.,0.));
#32218=CARTESIAN_POINT('',(26.251410108095,-2.36841946563064,0.00070651602448273));
#32219=CARTESIAN_POINT('',(26.448589891905,-2.37287786906969,-0.00183021142759643));
#32220=CARTESIAN_POINT('',(20.751410108095,-2.37175,-2.19152050672682E-14));
#32221=CARTESIAN_POINT('Ctrl Pts',(26.251410108095,-2.36841946563064,0.000706516024482698));
#32222=CARTESIAN_POINT('Ctrl Pts',(26.2805629646172,-2.36721059622311,-0.435181594253511));
#32223=CARTESIAN_POINT('Ctrl Pts',(26.3616445527737,-2.04562220805805,-1.64915798041796));
#32224=CARTESIAN_POINT('Ctrl Pts',(26.4946548725642,-0.118205880943649,
-2.78328803637694));
#32225=CARTESIAN_POINT('Ctrl Pts',(26.6504410674669,2.24374527752018,-1.65114209849832));
#32226=CARTESIAN_POINT('Ctrl Pts',(26.8062272623694,2.62218547960889,0.940642828993458));
#32227=CARTESIAN_POINT('Ctrl Pts',(26.962013457272,0.682564848581893,2.70088362563495));
#32228=CARTESIAN_POINT('Ctrl Pts',(27.1104077391805,-1.73978919606127,2.10326100923035));
#32229=CARTESIAN_POINT('Ctrl Pts',(27.2068732894548,-2.36854612418603,0.660527222904082));
#32230=CARTESIAN_POINT('Ctrl Pts',(27.251410108095,-2.3737047785273,-0.00158991435897499));
#32231=CARTESIAN_POINT('Ctrl Pts',(26.448589891905,-2.37287786906969,-0.00183021142759631));
#32232=CARTESIAN_POINT('Ctrl Pts',(26.458057685058,-2.37407608454277,-0.142713245404422));
#32233=CARTESIAN_POINT('Ctrl Pts',(26.5194542098452,-2.29941387975957,-1.05504174939956));
#32234=CARTESIAN_POINT('Ctrl Pts',(26.6327794662666,-1.11937732072311,-2.55101230581224));
#32235=CARTESIAN_POINT('Ctrl Pts',(26.7885656611692,1.49234563926014,-2.35235220176952));
#32236=CARTESIAN_POINT('Ctrl Pts',(26.9443518560717,2.78481186300027,-0.0741754152063169));
#32237=CARTESIAN_POINT('Ctrl Pts',(27.1001380509743,1.61544610555625,2.26958439782059));
#32238=CARTESIAN_POINT('Ctrl Pts',(27.2559242458769,-0.981988199781967,
2.60696950467868));
#32239=CARTESIAN_POINT('Ctrl Pts',(27.3720748595205,-2.27136583806211,1.14028354082802));
#32240=CARTESIAN_POINT('Ctrl Pts',(27.4362967415298,-2.37326379675183,0.185127362247078));
#32241=CARTESIAN_POINT('Ctrl Pts',(27.448589891905,-2.37168592243517,0.00196235655545921));
#32242=CARTESIAN_POINT('Origin',(20.751410108095,0.,0.));
#32243=CARTESIAN_POINT('',(25.251410108095,-2.3753084392137,0.000258694431195401));
#32244=CARTESIAN_POINT('',(25.448589891905,-2.36879324508993,0.00112237171147556));
#32245=CARTESIAN_POINT('',(20.751410108095,-2.37175,-2.19152050672682E-14));
#32246=CARTESIAN_POINT('Ctrl Pts',(25.251410108095,-2.3753084392137,0.000258694431195337));
#32247=CARTESIAN_POINT('Ctrl Pts',(25.3023239081454,-2.37409943004349,-0.755309212134195));
#32248=CARTESIAN_POINT('Ctrl Pts',(25.40516643983,-1.58145089662375,-2.28369713756637));
#32249=CARTESIAN_POINT('Ctrl Pts',(25.5599377031489,1.00151402983497,-2.59954499634369));
#32250=CARTESIAN_POINT('Ctrl Pts',(25.7157238980514,2.71606048046896,-0.619419004365017));
#32251=CARTESIAN_POINT('Ctrl Pts',(25.871510092954,2.02956013022766,1.90828459992846));
#32252=CARTESIAN_POINT('Ctrl Pts',(26.0272962878565,-0.451108261023179,
2.74902998834288));
#32253=CARTESIAN_POINT('Ctrl Pts',(26.1539296262369,-2.14339859605789,1.45702209482582));
#32254=CARTESIAN_POINT('Ctrl Pts',(26.228634232983,-2.36936390339549,0.341247181564567));
#32255=CARTESIAN_POINT('Ctrl Pts',(26.251410108095,-2.36841946563064,0.000706516024482698));
#32256=CARTESIAN_POINT('Ctrl Pts',(25.448589891905,-2.36879324508993,0.00112237171147545));
#32257=CARTESIAN_POINT('Ctrl Pts',(25.4798186285862,-2.36671530637589,-0.465618741150741));
#32258=CARTESIAN_POINT('Ctrl Pts',(25.5629760969016,-2.01029292083154,-1.71140950661792));
#32259=CARTESIAN_POINT('Ctrl Pts',(25.6980622968511,-0.00923482980258066,
-2.78578202961156));
#32260=CARTESIAN_POINT('Ctrl Pts',(25.8538484917537,2.30662002902024,-1.5621045377548));
#32261=CARTESIAN_POINT('Ctrl Pts',(26.0096346866563,2.58338094683827,1.04250164542461));
#32262=CARTESIAN_POINT('Ctrl Pts',(26.1654208815589,0.576386046271133,2.72551762147395));
#32263=CARTESIAN_POINT('Ctrl Pts',(26.3117392833084,-1.7872040174662,2.04327206314306));
#32264=CARTESIAN_POINT('Ctrl Pts',(26.4061289534238,-2.36750414019038,0.629998741958249));
#32265=CARTESIAN_POINT('Ctrl Pts',(26.448589891905,-2.37287786906969,-0.00183021142759631));
#32266=CARTESIAN_POINT('Origin',(20.751410108095,0.,0.));
#32267=CARTESIAN_POINT('',(24.251410108095,-2.36878253894032,-0.00111285785031767));
#32268=CARTESIAN_POINT('',(24.448589891905,-2.37530525058753,-0.000270455844553485));
#32269=CARTESIAN_POINT('',(20.751410108095,-2.37175,-2.19152050672682E-14));
#32270=CARTESIAN_POINT('Ctrl Pts',(24.251410108095,-2.36878253894032,-0.00111285785031799));
#32271=CARTESIAN_POINT('Ctrl Pts',(24.2721561200394,-2.37015216879397,-0.311184351495253));
#32272=CARTESIAN_POINT('Ctrl Pts',(24.344830863618,-2.17125111101719,-1.39570012081226));
#32273=CARTESIAN_POINT('Ctrl Pts',(24.4694343388309,-0.555935374140417,
-2.72976005070651));
#32274=CARTESIAN_POINT('Ctrl Pts',(24.6252205337334,1.95507743201704,-1.9845249725212));
#32275=CARTESIAN_POINT('Ctrl Pts',(24.781006728636,2.73776715706389,0.51506952434679));
#32276=CARTESIAN_POINT('Ctrl Pts',(24.9367929235385,1.10022053207099,2.55933153003611));
#32277=CARTESIAN_POINT('Ctrl Pts',(25.0925791184411,-1.50994080113541,2.3410988233723));
#32278=CARTESIAN_POINT('Ctrl Pts',(25.1974515132933,-2.36848045691257,0.800989302251748));
#32279=CARTESIAN_POINT('Ctrl Pts',(25.2503951765112,-2.37533253997991,0.0153204209432519));
#32280=CARTESIAN_POINT('Ctrl Pts',(25.251410108095,-2.3753084392137,0.000258694431195337));
#32281=CARTESIAN_POINT('Ctrl Pts',(24.448589891905,-2.37530525058753,-0.000270455844553585));
#32282=CARTESIAN_POINT('Ctrl Pts',(24.4496508404802,-2.37533152137686,-0.0160151494332644));
#32283=CARTESIAN_POINT('Ctrl Pts',(24.5026405206896,-2.36816253880158,-0.802368302582885));
#32284=CARTESIAN_POINT('Ctrl Pts',(24.6075589325332,-1.50790971480175,-2.34240766296688));
#32285=CARTESIAN_POINT('Ctrl Pts',(24.7633451274357,1.10244025446093,-2.55837695905924));
#32286=CARTESIAN_POINT('Ctrl Pts',(24.9191313223383,2.738213197235,-0.512694142435889));
#32287=CARTESIAN_POINT('Ctrl Pts',(25.0749175172409,1.95335583875086,1.98621940187114));
#32288=CARTESIAN_POINT('Ctrl Pts',(25.2307037121435,-0.558303519624818,
2.72927902174966));
#32289=CARTESIAN_POINT('Ctrl Pts',(25.3552611703648,-2.1718644533066,1.39430717464036));
#32290=CARTESIAN_POINT('Ctrl Pts',(25.427889896952,-2.3701706085527,0.310502119577585));
#32291=CARTESIAN_POINT('Ctrl Pts',(25.448589891905,-2.36879324508993,0.00112237171147545));
#32292=CARTESIAN_POINT('Origin',(20.751410108095,0.,0.));
#32293=CARTESIAN_POINT('',(23.251410108095,-2.37286196769524,0.00195470876282933));
#32294=CARTESIAN_POINT('',(23.448589891905,-2.36840991602323,-0.000688909241090413));
#32295=CARTESIAN_POINT('',(20.751410108095,-2.37175,-2.19152050672682E-14));
#32296=CARTESIAN_POINT('Ctrl Pts',(23.251410108095,-2.37286196769524,0.00195470876282933));
#32297=CARTESIAN_POINT('Ctrl Pts',(23.2939170635676,-2.36748782224901,-0.63054249811266));
#32298=CARTESIAN_POINT('Ctrl Pts',(23.3883527506744,-1.78622433682909,-2.0447933718034));
#32299=CARTESIAN_POINT('Ctrl Pts',(23.5347171694154,0.578777876478422,-2.72491209158622));
#32300=CARTESIAN_POINT('Ctrl Pts',(23.690503364318,2.58426961230329,-1.04031325744919));
#32301=CARTESIAN_POINT('Ctrl Pts',(23.8462895592206,2.30527110614996,1.56413143458517));
#32302=CARTESIAN_POINT('Ctrl Pts',(24.0020757541231,-0.0116548982896913,
2.78575885508703));
#32303=CARTESIAN_POINT('Ctrl Pts',(24.1371159370813,-2.01109387345396,1.71003568372357));
#32304=CARTESIAN_POINT('Ctrl Pts',(24.2202273884052,-2.36672388863589,0.464946474228187));
#32305=CARTESIAN_POINT('Ctrl Pts',(24.251410108095,-2.36878253894032,-0.00111285785031799));
#32306=CARTESIAN_POINT('Ctrl Pts',(23.448589891905,-2.36840991602323,-0.000688909241090621));
#32307=CARTESIAN_POINT('Ctrl Pts',(23.4714117840084,-2.36934544116764,-0.341925176311226));
#32308=CARTESIAN_POINT('Ctrl Pts',(23.546162407746,-2.1427579711721,-1.4584301293813));
#32309=CARTESIAN_POINT('Ctrl Pts',(23.6728417631177,-0.448717754286641,
-2.7494077907476));
#32310=CARTESIAN_POINT('Ctrl Pts',(23.8286279580203,2.03121191157331,-1.90653025915409));
#32311=CARTESIAN_POINT('Ctrl Pts',(23.9844141529229,2.7155240921129,0.621778103251025));
#32312=CARTESIAN_POINT('Ctrl Pts',(24.1402003478255,0.99925818313602,2.60041140430209));
#32313=CARTESIAN_POINT('Ctrl Pts',(24.2949255941528,-1.58266314056555,2.28242030819309));
#32314=CARTESIAN_POINT('Ctrl Pts',(24.397722108846,-2.37404568264673,0.754617836129284));
#32315=CARTESIAN_POINT('Ctrl Pts',(24.448589891905,-2.37530525058753,-0.000270455844553585));
#32316=CARTESIAN_POINT('Origin',(28.658,3.51939854619125E-16,0.));
#32317=CARTESIAN_POINT('',(28.658,0.261701021631923,2.93033728012268));
#32318=CARTESIAN_POINT('Ctrl Pts',(28.658,1.97801633036407,-1.31405326343373));
#32319=CARTESIAN_POINT('Ctrl Pts',(28.658,2.03588898944105,-1.24667939648802));
#32320=CARTESIAN_POINT('Ctrl Pts',(28.658,2.08963193546089,-1.17612088642746));
#32321=CARTESIAN_POINT('Ctrl Pts',(28.658,2.13887158382065,-1.10263113258862));
#32322=CARTESIAN_POINT('Ctrl Pts',(28.658,2.18456211831364,-1.03443840082659));
#32323=CARTESIAN_POINT('Ctrl Pts',(28.658,2.22637624274382,-0.963721068181632));
#32324=CARTESIAN_POINT('Ctrl Pts',(28.658,2.26436271250385,-0.890837075703206));
#32325=CARTESIAN_POINT('Ctrl Pts',(28.658,2.28264974318524,-0.855750061430627));
#32326=CARTESIAN_POINT('Ctrl Pts',(28.658,2.30004915173243,-0.82016034017639));
#32327=CARTESIAN_POINT('Ctrl Pts',(28.658,2.31656323187619,-0.784105041467371));
#32328=CARTESIAN_POINT('Ctrl Pts',(28.658,2.32355794425549,-0.768833440383695));
#32329=CARTESIAN_POINT('Ctrl Pts',(28.658,2.33039049782105,-0.75348540938221));
#32330=CARTESIAN_POINT('Ctrl Pts',(28.658,2.33705928183326,-0.738069100523836));
#32331=CARTESIAN_POINT('Ctrl Pts',(28.658,2.37145800155582,-0.658549163065291));
#32332=CARTESIAN_POINT('Ctrl Pts',(28.658,2.40152187518264,-0.577174196683355));
#32333=CARTESIAN_POINT('Ctrl Pts',(28.658,2.42731660870621,-0.494358545755739));
#32334=CARTESIAN_POINT('Ctrl Pts',(28.658,2.44988700053934,-0.421894851194075));
#32335=CARTESIAN_POINT('Ctrl Pts',(28.658,2.4691883185794,-0.348327044796147));
#32336=CARTESIAN_POINT('Ctrl Pts',(28.658,2.48523726885309,-0.273910862226402));
#32337=CARTESIAN_POINT('Ctrl Pts',(28.658,2.49043040451315,-0.249831198148779));
#32338=CARTESIAN_POINT('Ctrl Pts',(28.658,2.49528279533436,-0.225662577407877));
#32339=CARTESIAN_POINT('Ctrl Pts',(28.658,2.49979440405724,-0.20141333897661));
#32340=CARTESIAN_POINT('Ctrl Pts',(28.658,2.50272209611502,-0.185677421452916));
#32341=CARTESIAN_POINT('Ctrl Pts',(28.658,2.505506277858,-0.169907552756416));
#32342=CARTESIAN_POINT('Ctrl Pts',(28.658,2.50814687055771,-0.154105984441464));
#32343=CARTESIAN_POINT('Ctrl Pts',(28.658,2.51064326407261,-0.139167318333947));
#32344=CARTESIAN_POINT('Ctrl Pts',(28.658,2.51300962758955,-0.124210424344307));
#32345=CARTESIAN_POINT('Ctrl Pts',(28.658,2.51524622665656,-0.109238388801175));
#32346=CARTESIAN_POINT('Ctrl Pts',(28.658,2.52832241473202,-0.0217049745552181));
#32347=CARTESIAN_POINT('Ctrl Pts',(28.658,2.53696838029571,0.0663543248777591));
#32348=CARTESIAN_POINT('Ctrl Pts',(28.658,2.54124508921826,0.154537449743878));
#32349=CARTESIAN_POINT('Ctrl Pts',(28.658,2.54559508066862,0.244231615556881));
#32350=CARTESIAN_POINT('Ctrl Pts',(28.658,2.54542512050437,0.334054780156729));
#32351=CARTESIAN_POINT('Ctrl Pts',(28.658,2.54075262893098,0.423610145989604));
#32352=CARTESIAN_POINT('Ctrl Pts',(28.658,2.53686690572889,0.498085906388921));
#32353=CARTESIAN_POINT('Ctrl Pts',(28.658,2.52986651205561,0.572377218538135));
#32354=CARTESIAN_POINT('Ctrl Pts',(28.658,2.51973513979424,0.646262353103663));
#32355=CARTESIAN_POINT('Ctrl Pts',(28.658,2.51206070500465,0.702229761319919));
#32356=CARTESIAN_POINT('Ctrl Pts',(28.658,2.50258925346803,0.757964265454546));
#32357=CARTESIAN_POINT('Ctrl Pts',(28.658,2.4913040926272,0.813369424344011));
#32358=CARTESIAN_POINT('Ctrl Pts',(28.658,2.48766360830947,0.831242595573295));
#32359=CARTESIAN_POINT('Ctrl Pts',(28.658,2.483833274489,0.849085598142948));
#32360=CARTESIAN_POINT('Ctrl Pts',(28.658,2.4798188815792,0.866867679946036));
#32361=CARTESIAN_POINT('Ctrl Pts',(28.658,2.45941681290693,0.957240312180452));
#32362=CARTESIAN_POINT('Ctrl Pts',(28.658,2.43424071557649,1.04616757295001));
#32363=CARTESIAN_POINT('Ctrl Pts',(28.658,2.40432126657836,1.13323420516507));
#32364=CARTESIAN_POINT('Ctrl Pts',(28.658,2.38610167626726,1.18625384362247));
#32365=CARTESIAN_POINT('Ctrl Pts',(28.658,2.3661221590081,1.23858386635697));
#32366=CARTESIAN_POINT('Ctrl Pts',(28.658,2.34438027030047,1.29013186517359));
#32367=CARTESIAN_POINT('Ctrl Pts',(28.658,2.30980500483014,1.37210660837625));
#32368=CARTESIAN_POINT('Ctrl Pts',(28.658,2.27077563476682,1.45210464318559));
#32369=CARTESIAN_POINT('Ctrl Pts',(28.658,2.22760963761098,1.52996848770481));
#32370=CARTESIAN_POINT('Ctrl Pts',(28.658,2.20262999297066,1.57502736030302));
#32371=CARTESIAN_POINT('Ctrl Pts',(28.658,2.17626409255244,1.61937133560154));
#32372=CARTESIAN_POINT('Ctrl Pts',(28.658,2.14856603599913,1.66296748678073));
#32373=CARTESIAN_POINT('Ctrl Pts',(28.658,2.1288093227664,1.69406413268585));
#32374=CARTESIAN_POINT('Ctrl Pts',(28.658,2.10837472156678,1.72478026212631));
#32375=CARTESIAN_POINT('Ctrl Pts',(28.658,2.0872803454754,1.75510318279917));
#32376=CARTESIAN_POINT('Ctrl Pts',(28.658,2.07669314170718,1.77032216527205));
#32377=CARTESIAN_POINT('Ctrl Pts',(28.658,2.06593715859879,1.78544543077647));
#32378=CARTESIAN_POINT('Ctrl Pts',(28.658,2.05503140742641,1.80044869555866));
#32379=CARTESIAN_POINT('Ctrl Pts',(28.658,2.00068115281266,1.87521945165428));
#32380=CARTESIAN_POINT('Ctrl Pts',(28.658,1.94254510232413,1.9471157067966));
#32381=CARTESIAN_POINT('Ctrl Pts',(28.658,1.88099648476523,2.01598109009273));
#32382=CARTESIAN_POINT('Ctrl Pts',(28.658,1.81824029970113,2.08619759389164));
#32383=CARTESIAN_POINT('Ctrl Pts',(28.658,1.75193589590128,2.15326379417956));
#32384=CARTESIAN_POINT('Ctrl Pts',(28.658,1.68242589079217,2.21699709023191));
#32385=CARTESIAN_POINT('Ctrl Pts',(28.658,1.61227576386633,2.28131731003994));
#32386=CARTESIAN_POINT('Ctrl Pts',(28.658,1.53886014435481,2.34224366390707));
#32387=CARTESIAN_POINT('Ctrl Pts',(28.658,1.46248554098919,2.39956107936614));
#32388=CARTESIAN_POINT('Ctrl Pts',(28.658,1.41833873564515,2.43269226004124));
#32389=CARTESIAN_POINT('Ctrl Pts',(28.658,1.37320247880795,2.46461706605157));
#32390=CARTESIAN_POINT('Ctrl Pts',(28.658,1.32713029596024,2.49528840587952));
#32391=CARTESIAN_POINT('Ctrl Pts',(28.658,1.31488967467329,2.5034372764559));
#32392=CARTESIAN_POINT('Ctrl Pts',(28.658,1.30258075027275,2.511499067118));
#32393=CARTESIAN_POINT('Ctrl Pts',(28.658,1.29021178873854,2.51946814645669));
#32394=CARTESIAN_POINT('Ctrl Pts',(28.658,1.20764107863156,2.57266683561706));
#32395=CARTESIAN_POINT('Ctrl Pts',(28.658,1.12259640491928,2.62161093215467));
#32396=CARTESIAN_POINT('Ctrl Pts',(28.658,1.03544610319146,2.66611476104981));
#32397=CARTESIAN_POINT('Ctrl Pts',(28.658,0.947976267227596,2.71078176203599));
#32398=CARTESIAN_POINT('Ctrl Pts',(28.658,0.858384645681997,2.75097657191429));
#32399=CARTESIAN_POINT('Ctrl Pts',(28.658,0.76700170558157,2.7864795973746));
#32400=CARTESIAN_POINT('Ctrl Pts',(28.658,0.677259469945933,2.82134519562669));
#32401=CARTESIAN_POINT('Ctrl Pts',(28.658,0.585788889330719,2.85168650745828));
#32402=CARTESIAN_POINT('Ctrl Pts',(28.658,0.492873620233273,2.87725594522238));
#32403=CARTESIAN_POINT('Ctrl Pts',(28.658,0.416738026937611,2.89820776867741));
#32404=CARTESIAN_POINT('Ctrl Pts',(28.658,0.339631723233453,2.91595505282006));
#32405=CARTESIAN_POINT('Ctrl Pts',(28.658,0.261701021631923,2.93033728012268));
#32406=CARTESIAN_POINT('',(28.658,-2.942,-3.60291088309151E-16));
#32407=CARTESIAN_POINT('Origin',(28.658,0.,0.));
#32408=CARTESIAN_POINT('',(28.658,-2.15060832247059,2.01293848078683));
#32409=CARTESIAN_POINT('Origin',(28.658,0.,0.));
#32410=CARTESIAN_POINT('Ctrl Pts',(28.658,-2.15060832247059,2.01293848078683));
#32411=CARTESIAN_POINT('Ctrl Pts',(28.658,-2.20971109593349,1.93767297749437));
#32412=CARTESIAN_POINT('Ctrl Pts',(28.658,-2.26481658708665,1.85956683039048));
#32413=CARTESIAN_POINT('Ctrl Pts',(28.658,-2.31558252285751,1.77874869425101));
#32414=CARTESIAN_POINT('Ctrl Pts',(28.658,-2.32237888851895,1.76792904526908));
#32415=CARTESIAN_POINT('Ctrl Pts',(28.658,-2.32909740761893,1.75706075632002));
#32416=CARTESIAN_POINT('Ctrl Pts',(28.658,-2.33573719302841,1.74614410673189));
#32417=CARTESIAN_POINT('Ctrl Pts',(28.658,-2.38668022372525,1.66238730123612));
#32418=CARTESIAN_POINT('Ctrl Pts',(28.658,-2.43299277513564,1.57578453084994));
#32419=CARTESIAN_POINT('Ctrl Pts',(28.658,-2.47464052311135,1.48675406675739));
#32420=CARTESIAN_POINT('Ctrl Pts',(28.658,-2.48689377831249,1.46056026156441));
#32421=CARTESIAN_POINT('Ctrl Pts',(28.658,-2.49874290551813,1.43415626299096));
#32422=CARTESIAN_POINT('Ctrl Pts',(28.658,-2.51018618118443,1.40755265714468));
#32423=CARTESIAN_POINT('Ctrl Pts',(28.658,-2.51771390631931,1.39005201849476));
#32424=CARTESIAN_POINT('Ctrl Pts',(28.658,-2.52506599547472,1.37246500180567));
#32425=CARTESIAN_POINT('Ctrl Pts',(28.658,-2.53224186714647,1.35479462666926));
#32426=CARTESIAN_POINT('Ctrl Pts',(28.658,-2.53962113906836,1.33662338433687));
#32427=CARTESIAN_POINT('Ctrl Pts',(28.658,-2.54681097419375,1.31837145371668));
#32428=CARTESIAN_POINT('Ctrl Pts',(28.658,-2.55380852110088,1.30004960134548));
#32429=CARTESIAN_POINT('Ctrl Pts',(28.658,-2.58844585274772,1.20935780815165));
#32430=CARTESIAN_POINT('Ctrl Pts',(28.658,-2.61839882158235,1.11689744862561));
#32431=CARTESIAN_POINT('Ctrl Pts',(28.658,-2.64365122411707,1.02308128352135));
#32432=CARTESIAN_POINT('Ctrl Pts',(28.658,-2.66475485704852,0.944678370821319));
#32433=CARTESIAN_POINT('Ctrl Pts',(28.658,-2.68257463739759,0.865327992912511));
#32434=CARTESIAN_POINT('Ctrl Pts',(28.658,-2.69707318068004,0.785271122320479));
#32435=CARTESIAN_POINT('Ctrl Pts',(28.658,-2.70352672731022,0.749636456315314));
#32436=CARTESIAN_POINT('Ctrl Pts',(28.658,-2.70932190569519,0.713861857690371));
#32437=CARTESIAN_POINT('Ctrl Pts',(28.658,-2.7144538141254,0.677968940347287));
#32438=CARTESIAN_POINT('Ctrl Pts',(28.658,-2.71700175179471,0.660148490624957));
#32439=CARTESIAN_POINT('Ctrl Pts',(28.658,-2.71938617708855,0.642298879916618));
#32440=CARTESIAN_POINT('Ctrl Pts',(28.658,-2.72160640006766,0.624422786102583));
#32441=CARTESIAN_POINT('Ctrl Pts',(28.658,-2.72363648596765,0.608077578283332));
#32442=CARTESIAN_POINT('Ctrl Pts',(28.658,-2.72552824448812,0.591718366592941));
#32443=CARTESIAN_POINT('Ctrl Pts',(28.658,-2.72728098621858,0.575353162719347));
#32444=CARTESIAN_POINT('Ctrl Pts',(28.658,-2.73739781604062,0.480893163442538));
#32445=CARTESIAN_POINT('Ctrl Pts',(28.658,-2.74289532062776,0.386169908251331));
#32446=CARTESIAN_POINT('Ctrl Pts',(28.658,-2.7437548509834,0.291566670300918));
#32447=CARTESIAN_POINT('Ctrl Pts',(28.658,-2.74460687110618,0.197790037650447));
#32448=CARTESIAN_POINT('Ctrl Pts',(28.658,-2.74090146504082,0.104130391083328));
#32449=CARTESIAN_POINT('Ctrl Pts',(28.658,-2.73257054458709,0.010970921487669));
#32450=CARTESIAN_POINT('Ctrl Pts',(28.658,-2.72570835794339,-0.065764617105541));
#32451=CARTESIAN_POINT('Ctrl Pts',(28.658,-2.7157069180874,-0.142160847495387));
#32452=CARTESIAN_POINT('Ctrl Pts',(28.658,-2.70250334697467,-0.217991837109981));
#32453=CARTESIAN_POINT('Ctrl Pts',(28.658,-2.69260066864013,-0.274865079320927));
#32454=CARTESIAN_POINT('Ctrl Pts',(28.658,-2.68089633000001,-0.331420179713332));
#32455=CARTESIAN_POINT('Ctrl Pts',(28.658,-2.66735565981843,-0.387555995282867));
#32456=CARTESIAN_POINT('Ctrl Pts',(28.658,-2.66394701524533,-0.401687278338419));
#32457=CARTESIAN_POINT('Ctrl Pts',(28.658,-2.66042196824992,-0.415791962607326));
#32458=CARTESIAN_POINT('Ctrl Pts',(28.658,-2.65677989678547,-0.429868374047563));
#32459=CARTESIAN_POINT('Ctrl Pts',(28.658,-2.65341425236481,-0.442876409746268));
#32460=CARTESIAN_POINT('Ctrl Pts',(28.658,-2.64994974372578,-0.455856001451419));
#32461=CARTESIAN_POINT('Ctrl Pts',(28.658,-2.64638824974718,-0.468798346640149));
#32462=CARTESIAN_POINT('Ctrl Pts',(28.658,-2.62270732724449,-0.554853994988378));
#32463=CARTESIAN_POINT('Ctrl Pts',(28.658,-2.59471590580757,-0.639367325882882));
#32464=CARTESIAN_POINT('Ctrl Pts',(28.658,-2.56235842010114,-0.7219999177347));
#32465=CARTESIAN_POINT('Ctrl Pts',(28.658,-2.54209052173618,-0.773758851926326));
#32466=CARTESIAN_POINT('Ctrl Pts',(28.658,-2.52010870092681,-0.824779529231049));
#32467=CARTESIAN_POINT('Ctrl Pts',(28.658,-2.4963902536118,-0.874973476494181));
#32468=CARTESIAN_POINT('Ctrl Pts',(28.658,-2.45769064340973,-0.956871172738262));
#32469=CARTESIAN_POINT('Ctrl Pts',(28.658,-2.41436920801051,-1.03657008506992));
#32470=CARTESIAN_POINT('Ctrl Pts',(28.658,-2.36672566050128,-1.11382437417113));
#32471=CARTESIAN_POINT('Ctrl Pts',(28.658,-2.31891811374559,-1.19134458900331));
#32472=CARTESIAN_POINT('Ctrl Pts',(28.658,-2.2667577640464,-1.26640389984806));
#32473=CARTESIAN_POINT('Ctrl Pts',(28.658,-2.21051982316866,-1.33870955140761));
#32474=CARTESIAN_POINT('Ctrl Pts',(28.658,-2.20189537756213,-1.34979808255201));
#32475=CARTESIAN_POINT('Ctrl Pts',(28.658,-2.19318006476582,-1.36081520380594));
#32476=CARTESIAN_POINT('Ctrl Pts',(28.658,-2.18437794934293,-1.37175665419369));
#32477=CARTESIAN_POINT('Ctrl Pts',(28.658,-2.12879717302225,-1.4408462170326));
#32478=CARTESIAN_POINT('Ctrl Pts',(28.658,-2.06972321612038,-1.50696694812369));
#32479=CARTESIAN_POINT('Ctrl Pts',(28.658,-2.0074651266359,-1.5699147697608));
#32480=CARTESIAN_POINT('Ctrl Pts',(28.658,-1.9452667315866,-1.63280223563227));
#32481=CARTESIAN_POINT('Ctrl Pts',(28.658,-1.87988940823054,-1.69252336443322));
#32482=CARTESIAN_POINT('Ctrl Pts',(28.658,-1.81161260297583,-1.74883157744085));
#32483=CARTESIAN_POINT('Ctrl Pts',(28.658,-1.74439799581986,-1.8042637905159));
#32484=CARTESIAN_POINT('Ctrl Pts',(28.658,-1.67437256396589,-1.85638878596463));
#32485=CARTESIAN_POINT('Ctrl Pts',(28.658,-1.60178815117267,-1.9049236123197));
#32486=CARTESIAN_POINT('Ctrl Pts',(28.658,-1.57702435474135,-1.92148235425112));
#32487=CARTESIAN_POINT('Ctrl Pts',(28.658,-1.55196262566561,-1.93762276924518));
#32488=CARTESIAN_POINT('Ctrl Pts',(28.658,-1.52661283080042,-1.95333221692257));
#32489=CARTESIAN_POINT('Ctrl Pts',(28.658,-1.5105418481757,-1.96329151884236));
#32490=CARTESIAN_POINT('Ctrl Pts',(28.658,-1.49435508656289,-1.97307759307412));
#32491=CARTESIAN_POINT('Ctrl Pts',(28.658,-1.47805506249159,-1.98268706081389));
#32492=CARTESIAN_POINT('Ctrl Pts',(28.658,-1.46641505727283,-1.98954927489106));
#32493=CARTESIAN_POINT('Ctrl Pts',(28.658,-1.45472491992427,-1.99631691153973));
#32494=CARTESIAN_POINT('Ctrl Pts',(28.658,-1.44298829166971,-2.00298769190301));
#32495=CARTESIAN_POINT('Ctrl Pts',(28.658,-1.3688399031693,-2.04513161972017));
#32496=CARTESIAN_POINT('Ctrl Pts',(28.658,-1.2928037819447,-2.08343336979007));
#32497=CARTESIAN_POINT('Ctrl Pts',(28.658,-1.21513616067108,-2.11767523333238));
#32498=CARTESIAN_POINT('Ctrl Pts',(28.658,-1.13866984115548,-2.15138747062637));
#32499=CARTESIAN_POINT('Ctrl Pts',(28.658,-1.06062131430581,-2.18116469203935));
#32500=CARTESIAN_POINT('Ctrl Pts',(28.658,-0.981226066391064,-2.20675022144869));
#32501=CARTESIAN_POINT('Ctrl Pts',(28.658,-0.904293774038269,-2.23154205068555));
#32502=CARTESIAN_POINT('Ctrl Pts',(28.658,-0.826096380893346,-2.25239828191146));
#32503=CARTESIAN_POINT('Ctrl Pts',(28.658,-0.74684990431363,-2.26903704779655));
#32504=CARTESIAN_POINT('Ctrl Pts',(28.658,-0.69773198312443,-2.27934995540711));
#32505=CARTESIAN_POINT('Ctrl Pts',(28.658,-0.648211111266871,-2.28804169467426));
#32506=CARTESIAN_POINT('Ctrl Pts',(28.658,-0.598340649004787,-2.29503519150547));
#32507=CARTESIAN_POINT('Ctrl Pts',(22.2707660089946,-1.03908919352505,2.13201587949046));
#32508=CARTESIAN_POINT('Ctrl Pts',(22.3226947406288,-1.73471873725821,1.79298409809367));
#32509=CARTESIAN_POINT('Ctrl Pts',(22.4265522038972,-2.75780127841751,0.387620901480232));
#32510=CARTESIAN_POINT('Ctrl Pts',(22.5823383987998,-1.85932621210726,-2.07658872801938));
#32511=CARTESIAN_POINT('Ctrl Pts',(22.7381245937023,0.68524861492584,-2.6995454694093));
#32512=CARTESIAN_POINT('Ctrl Pts',(22.8939107886049,2.62282735660906,-0.938746401795666));
#32513=CARTESIAN_POINT('Ctrl Pts',(23.0496969835074,2.24240074214882,1.65328021767869));
#32514=CARTESIAN_POINT('Ctrl Pts',(23.2054831784101,-0.120664916242889,
2.78308709983206));
#32515=CARTESIAN_POINT('Ctrl Pts',(23.3612693733126,-2.37689989423139,1.45294520051045));
#32516=CARTESIAN_POINT('Ctrl Pts',(23.5170555682152,-2.53199390158006,-1.16180500434049));
#32517=CARTESIAN_POINT('Ctrl Pts',(23.6728417631177,-0.448717754286641,
-2.7494077907476));
#32518=CARTESIAN_POINT('Ctrl Pts',(23.8286279580203,2.03121191157331,-1.90653025915409));
#32519=CARTESIAN_POINT('Ctrl Pts',(23.9844141529229,2.7155240921129,0.621778103251025));
#32520=CARTESIAN_POINT('Ctrl Pts',(24.1402003478255,0.99925818313602,2.60041140430209));
#32521=CARTESIAN_POINT('Ctrl Pts',(24.295986542728,-1.60036733438438,2.28023984825943));
#32522=CARTESIAN_POINT('Ctrl Pts',(24.4517727376306,-2.78524046876828,-0.0557082387313367));
#32523=CARTESIAN_POINT('Ctrl Pts',(24.6075589325332,-1.50790971480175,-2.34240766296688));
#32524=CARTESIAN_POINT('Ctrl Pts',(24.7633451274357,1.10244025446093,-2.55837695905924));
#32525=CARTESIAN_POINT('Ctrl Pts',(24.9191313223383,2.738213197235,-0.512694142435889));
#32526=CARTESIAN_POINT('Ctrl Pts',(25.0749175172409,1.95335583875086,1.98621940187114));
#32527=CARTESIAN_POINT('Ctrl Pts',(25.2307037121435,-0.558303519624818,
2.72927902174966));
#32528=CARTESIAN_POINT('Ctrl Pts',(25.386489907046,-2.5764124445433,1.0596063475242));
#32529=CARTESIAN_POINT('Ctrl Pts',(25.5422761019486,-2.31692596255169,-1.54677754708461));
#32530=CARTESIAN_POINT('Ctrl Pts',(25.6980622968511,-0.00923482980258066,
-2.78578202961156));
#32531=CARTESIAN_POINT('Ctrl Pts',(25.8538484917537,2.30662002902024,-1.5621045377548));
#32532=CARTESIAN_POINT('Ctrl Pts',(26.0096346866563,2.58338094683827,1.04250164542461));
#32533=CARTESIAN_POINT('Ctrl Pts',(26.1654208815589,0.576386046271133,2.72551762147395));
#32534=CARTESIAN_POINT('Ctrl Pts',(26.3212070764614,-1.94014432814736,1.99912614746469));
#32535=CARTESIAN_POINT('Ctrl Pts',(26.476993271364,-2.7415523872825,-0.494528446616266));
#32536=CARTESIAN_POINT('Ctrl Pts',(26.6327794662666,-1.11937732072311,-2.55101230581224));
#32537=CARTESIAN_POINT('Ctrl Pts',(26.7885656611692,1.49234563926014,-2.35235220176952));
#32538=CARTESIAN_POINT('Ctrl Pts',(26.9443518560717,2.78481186300027,-0.0741754152063169));
#32539=CARTESIAN_POINT('Ctrl Pts',(27.1001380509743,1.61544610555625,2.26958439782059));
#32540=CARTESIAN_POINT('Ctrl Pts',(27.2559242458769,-0.981988199781967,
2.60696950467868));
#32541=CARTESIAN_POINT('Ctrl Pts',(27.4117104407795,-2.71135690270178,0.639787255203349));
#32542=CARTESIAN_POINT('Ctrl Pts',(27.567496635682,-2.04377823479325,-1.89305926739468));
#32543=CARTESIAN_POINT('Ctrl Pts',(27.7232828305846,0.430422244683163,-2.75224826615359));
#32544=CARTESIAN_POINT('Ctrl Pts',(27.8790690254871,2.52434834774427,-1.17871200290743));
#32545=CARTESIAN_POINT('Ctrl Pts',(28.0348552203897,2.38625876548845,1.43744121743837));
#32546=CARTESIAN_POINT('Ctrl Pts',(28.1906414152923,0.139550436043699,2.78166084946855));
#32547=CARTESIAN_POINT('Ctrl Pts',(28.3464276101949,-2.2322534987586,1.66923905587135));
#32548=CARTESIAN_POINT('Ctrl Pts',(28.5022138050974,-2.62724420518177,-0.923745495709923));
#32549=CARTESIAN_POINT('Ctrl Pts',(28.6060712683658,-1.34715978233134,-2.09980989479535));
#32550=CARTESIAN_POINT('Ctrl Pts',(28.658,-0.598340649004787,-2.29503519150547));
#32551=CARTESIAN_POINT('Ctrl Pts',(22.3805106726631,-1.12236674703443,2.3028857793927));
#32552=CARTESIAN_POINT('Ctrl Pts',(22.4324394042973,-1.87374735324802,1.93668237741455));
#32553=CARTESIAN_POINT('Ctrl Pts',(22.5362968675657,-2.97882459861252,0.418686685404777));
#32554=CARTESIAN_POINT('Ctrl Pts',(22.6920830624682,-2.00834146420018,-2.24301643219745));
#32555=CARTESIAN_POINT('Ctrl Pts',(22.8478692573708,0.740167700363659,-2.91589989180214));
#32556=CARTESIAN_POINT('Ctrl Pts',(23.0036554522733,2.83303322430258,-1.0139820063948));
#32557=CARTESIAN_POINT('Ctrl Pts',(23.1594416471759,2.42211741032076,1.78578196310313));
#32558=CARTESIAN_POINT('Ctrl Pts',(23.3152278420785,-0.130335576934711,
3.00613694610299));
#32559=CARTESIAN_POINT('Ctrl Pts',(23.4710140369811,-2.56739596459932,1.56939114416543));
#32560=CARTESIAN_POINT('Ctrl Pts',(23.6268002318836,-2.73491994386615,-1.25491758699396));
#32561=CARTESIAN_POINT('Ctrl Pts',(23.7825864267862,-0.484680130785283,
-2.96975841689198));
#32562=CARTESIAN_POINT('Ctrl Pts',(23.9383726216888,2.19400290171065,-2.0593286682448));
#32563=CARTESIAN_POINT('Ctrl Pts',(24.0941588165914,2.93315911737939,0.671610359795614));
#32564=CARTESIAN_POINT('Ctrl Pts',(24.2499450114939,1.07934348989732,2.80882075088911));
#32565=CARTESIAN_POINT('Ctrl Pts',(24.4057312063965,-1.72862838950299,2.46298912249013));
#32566=CARTESIAN_POINT('Ctrl Pts',(24.561517401299,-3.00846289627471,-0.0601729621263726));
#32567=CARTESIAN_POINT('Ctrl Pts',(24.7173035962016,-1.62876077623539,-2.53013936175565));
#32568=CARTESIAN_POINT('Ctrl Pts',(24.8730897911042,1.1907950635128,-2.76341746514174));
#32569=CARTESIAN_POINT('Ctrl Pts',(25.0288759860068,2.95766663537466,-0.553783891176143));
#32570=CARTESIAN_POINT('Ctrl Pts',(25.1846621809093,2.10990707265658,2.1454044781393));
#32571=CARTESIAN_POINT('Ctrl Pts',(25.3404483758119,-0.603048620930609,
2.94801643254376));
#32572=CARTESIAN_POINT('Ctrl Pts',(25.4962345707145,-2.78289840027231,1.14452824340639));
#32573=CARTESIAN_POINT('Ctrl Pts',(25.652020765617,-2.50261543658917,-1.67074366158866));
#32574=CARTESIAN_POINT('Ctrl Pts',(25.8078069605196,-0.00997495301609062,
-3.00904786038153));
#32575=CARTESIAN_POINT('Ctrl Pts',(25.9635931554222,2.49148353649345,-1.68729903023991));
#32576=CARTESIAN_POINT('Ctrl Pts',(26.1193793503248,2.79042539150775,1.12605268907077));
#32577=CARTESIAN_POINT('Ctrl Pts',(26.2751655452273,0.622580367326068,2.94395357574758));
#32578=CARTESIAN_POINT('Ctrl Pts',(26.4309517401299,-2.09563672871319,2.15934563175432));
#32579=CARTESIAN_POINT('Ctrl Pts',(26.5867379350324,-2.96127344400544,-0.534162310033983));
#32580=CARTESIAN_POINT('Ctrl Pts',(26.7425241299351,-1.20908954687713,-2.7554625735315));
#32581=CARTESIAN_POINT('Ctrl Pts',(26.8983103248376,1.61194932160273,-2.54088090322894));
#32582=CARTESIAN_POINT('Ctrl Pts',(27.0540965197402,3.0079999400005,-0.0801201860185042));
#32583=CARTESIAN_POINT('Ctrl Pts',(27.2098827146428,1.74491564516392,2.45147969353855));
#32584=CARTESIAN_POINT('Ctrl Pts',(27.3656689095453,-1.06068940788086,2.81590444864312));
#32585=CARTESIAN_POINT('Ctrl Pts',(27.5214551044479,-2.92865794957514,0.691062850899878));
#32586=CARTESIAN_POINT('Ctrl Pts',(27.6772412993505,-2.20757634988279,-2.04477804709066));
#32587=CARTESIAN_POINT('Ctrl Pts',(27.833027494253,0.464918331964785,-2.97282654151624));
#32588=CARTESIAN_POINT('Ctrl Pts',(27.9888136891556,2.72666163895697,-1.27317959289484));
#32589=CARTESIAN_POINT('Ctrl Pts',(28.1445998840582,2.57750490034244,1.55264459809882));
#32590=CARTESIAN_POINT('Ctrl Pts',(28.3003860789608,0.150734672177907,3.00459638924711));
#32591=CARTESIAN_POINT('Ctrl Pts',(28.4561722738633,-2.41115691854948,1.80301981854457));
#32592=CARTESIAN_POINT('Ctrl Pts',(28.6119584687659,-2.83780406014188,-0.997778856298598));
#32593=CARTESIAN_POINT('Ctrl Pts',(28.7158159320343,-1.45512757908823,-2.26809865379989));
#32594=CARTESIAN_POINT('Ctrl Pts',(28.7677446636685,-0.646294516415629,
-2.47897023496227));
#32595=CARTESIAN_POINT('Ctrl Pts',(22.4902553363315,-1.20564430054382,2.47375567929494));
#32596=CARTESIAN_POINT('Ctrl Pts',(22.5421840679657,-2.01277596923782,2.08038065673544));
#32597=CARTESIAN_POINT('Ctrl Pts',(22.6460415312341,-3.19984791880754,0.449752469329321));
#32598=CARTESIAN_POINT('Ctrl Pts',(22.8018277261367,-2.1573567162931,-2.40944413637552));
#32599=CARTESIAN_POINT('Ctrl Pts',(22.9576139210393,0.795086785801479,-3.13225431419499));
#32600=CARTESIAN_POINT('Ctrl Pts',(23.1134001159418,3.0432390919961,-1.08921761099393));
#32601=CARTESIAN_POINT('Ctrl Pts',(23.2691863108444,2.6018340784927,1.91828370852757));
#32602=CARTESIAN_POINT('Ctrl Pts',(23.4249725057469,-0.140006237626535,
3.22918679237392));
#32603=CARTESIAN_POINT('Ctrl Pts',(23.5807587006495,-2.75789203496725,1.68583708782041));
#32604=CARTESIAN_POINT('Ctrl Pts',(23.7365448955521,-2.93784598615223,-1.34803016964744));
#32605=CARTESIAN_POINT('Ctrl Pts',(23.8923310904547,-0.520642507283926,
-3.19010904303636));
#32606=CARTESIAN_POINT('Ctrl Pts',(24.0481172853572,2.35679389184798,-2.2121270773355));
#32607=CARTESIAN_POINT('Ctrl Pts',(24.2039034802598,3.15079414264587,0.721442616340202));
#32608=CARTESIAN_POINT('Ctrl Pts',(24.3596896751624,1.15942879665862,3.01723009747613));
#32609=CARTESIAN_POINT('Ctrl Pts',(24.515475870065,-1.8568894446216,2.64573839672082));
#32610=CARTESIAN_POINT('Ctrl Pts',(24.6712620649675,-3.23168532378114,-0.0646376855214102));
#32611=CARTESIAN_POINT('Ctrl Pts',(24.8270482598701,-1.74961183766903,-2.71787106054443));
#32612=CARTESIAN_POINT('Ctrl Pts',(24.9828344547727,1.27914987256467,-2.96845797122425));
#32613=CARTESIAN_POINT('Ctrl Pts',(25.1386206496752,3.17712007351433,-0.594873639916395));
#32614=CARTESIAN_POINT('Ctrl Pts',(25.2944068445778,2.26645830656231,2.30458955440746));
#32615=CARTESIAN_POINT('Ctrl Pts',(25.4501930394804,-0.647793722236402,
3.16675384333786));
#32616=CARTESIAN_POINT('Ctrl Pts',(25.6059792343829,-2.98938435600131,1.22945013928857));
#32617=CARTESIAN_POINT('Ctrl Pts',(25.7617654292856,-2.68830491062663,-1.79470977609272));
#32618=CARTESIAN_POINT('Ctrl Pts',(25.9175516241881,-0.0107150762296046,
-3.23231369115149));
#32619=CARTESIAN_POINT('Ctrl Pts',(26.0733378190907,2.67634704396667,-1.81249352272502));
#32620=CARTESIAN_POINT('Ctrl Pts',(26.2291240139932,2.99746983617723,1.20960373271694));
#32621=CARTESIAN_POINT('Ctrl Pts',(26.3849102088958,0.668774688381005,3.16238953002122));
#32622=CARTESIAN_POINT('Ctrl Pts',(26.5406964037984,-2.25112912927902,2.31956511604394));
#32623=CARTESIAN_POINT('Ctrl Pts',(26.6964825987009,-3.18099450072837,-0.573796173451701));
#32624=CARTESIAN_POINT('Ctrl Pts',(26.8522687936035,-1.29880177303115,-2.95991284125075));
#32625=CARTESIAN_POINT('Ctrl Pts',(27.0080549885061,1.73155300394531,-2.72940960468835));
#32626=CARTESIAN_POINT('Ctrl Pts',(27.1638411834086,3.23118801700073,-0.0860649568306912));
#32627=CARTESIAN_POINT('Ctrl Pts',(27.3196273783112,1.87438518477158,2.6333749892565));
#32628=CARTESIAN_POINT('Ctrl Pts',(27.4754135732138,-1.13939061597976,3.02483939260757));
#32629=CARTESIAN_POINT('Ctrl Pts',(27.6311997681164,-3.14595899644851,0.742338446596407));
#32630=CARTESIAN_POINT('Ctrl Pts',(27.7869859630189,-2.37137446497233,-2.19649682678664));
#32631=CARTESIAN_POINT('Ctrl Pts',(27.9427721579215,0.499414419246406,-3.19340481687888));
#32632=CARTESIAN_POINT('Ctrl Pts',(28.098558352824,2.92897493016967,-1.36764718288226));
#32633=CARTESIAN_POINT('Ctrl Pts',(28.2543445477267,2.76875103519641,1.66784797875926));
#32634=CARTESIAN_POINT('Ctrl Pts',(28.4101307426292,0.161918908312118,3.22753192902568));
#32635=CARTESIAN_POINT('Ctrl Pts',(28.5659169375318,-2.59006033834036,1.93680058121779));
#32636=CARTESIAN_POINT('Ctrl Pts',(28.7217031324344,-3.04836391510199,-1.07181221688727));
#32637=CARTESIAN_POINT('Ctrl Pts',(28.8255605957027,-1.56309537584512,-2.43638741280443));
#32638=CARTESIAN_POINT('Ctrl Pts',(28.8774893273369,-0.69424838382647,-2.66290527841906));
#32639=CARTESIAN_POINT('Ctrl Pts',(22.6,-1.2889218540532,2.64462557919719));
#32640=CARTESIAN_POINT('Ctrl Pts',(22.6519287316342,-2.15180458522763,2.22407893605632));
#32641=CARTESIAN_POINT('Ctrl Pts',(22.7557861949026,-3.42087123900255,0.480818253253867));
#32642=CARTESIAN_POINT('Ctrl Pts',(22.9115723898051,-2.30637196838603,-2.5758718405536));
#32643=CARTESIAN_POINT('Ctrl Pts',(23.0673585847077,0.850005871239299,-3.34860873658782));
#32644=CARTESIAN_POINT('Ctrl Pts',(23.2231447796103,3.25344495968962,-1.16445321559307));
#32645=CARTESIAN_POINT('Ctrl Pts',(23.3789309745129,2.78155074666463,2.05078545395201));
#32646=CARTESIAN_POINT('Ctrl Pts',(23.5347171694154,-0.149676898318359,
3.45223663864485));
#32647=CARTESIAN_POINT('Ctrl Pts',(23.690503364318,-2.94838810533518,1.80228303147539));
#32648=CARTESIAN_POINT('Ctrl Pts',(23.8462895592206,-3.14077202843831,-1.44114275230091));
#32649=CARTESIAN_POINT('Ctrl Pts',(24.0020757541232,-0.556604883782569,
-3.41045966918074));
#32650=CARTESIAN_POINT('Ctrl Pts',(24.1578619490257,2.51958488198532,-2.36492548642621));
#32651=CARTESIAN_POINT('Ctrl Pts',(24.3136481439283,3.36842916791236,0.77127487288479));
#32652=CARTESIAN_POINT('Ctrl Pts',(24.4694343388308,1.23951410341992,3.22563944406314));
#32653=CARTESIAN_POINT('Ctrl Pts',(24.6252205337334,-1.98515049974021,2.82848767095152));
#32654=CARTESIAN_POINT('Ctrl Pts',(24.781006728636,-3.45490775128757,-0.0691024089164465));
#32655=CARTESIAN_POINT('Ctrl Pts',(24.9367929235386,-1.87046289910267,-2.90560275933321));
#32656=CARTESIAN_POINT('Ctrl Pts',(25.0925791184411,1.36750468161654,-3.17349847730675));
#32657=CARTESIAN_POINT('Ctrl Pts',(25.2483653133437,3.39657351165399,-0.635963388656646));
#32658=CARTESIAN_POINT('Ctrl Pts',(25.4041515082463,2.42300954046803,2.46377463067561));
#32659=CARTESIAN_POINT('Ctrl Pts',(25.5599377031488,-0.692538823542196,
3.38549125413197));
#32660=CARTESIAN_POINT('Ctrl Pts',(25.7157238980514,-3.19587031173032,1.31437203517075));
#32661=CARTESIAN_POINT('Ctrl Pts',(25.871510092954,-2.87399438466411,-1.91867589059677));
#32662=CARTESIAN_POINT('Ctrl Pts',(26.0272962878565,-0.0114551994431134,
-3.45557952192146));
#32663=CARTESIAN_POINT('Ctrl Pts',(26.1830824827591,2.86121055143987,-1.93768801521013));
#32664=CARTESIAN_POINT('Ctrl Pts',(26.3388686776617,3.20451428084672,1.2931547763631));
#32665=CARTESIAN_POINT('Ctrl Pts',(26.4946548725642,0.714969009435938,3.38082548429487));
#32666=CARTESIAN_POINT('Ctrl Pts',(26.6504410674668,-2.40662152984485,2.47978460033357));
#32667=CARTESIAN_POINT('Ctrl Pts',(26.8062272623694,-3.4007155574513,-0.613430036869417));
#32668=CARTESIAN_POINT('Ctrl Pts',(26.962013457272,-1.38851399918516,-3.16436310897001));
#32669=CARTESIAN_POINT('Ctrl Pts',(27.1177996521745,1.8511566862879,-2.91793830614776));
#32670=CARTESIAN_POINT('Ctrl Pts',(27.2735858470772,3.45437609400096,-0.0920097276428782));
#32671=CARTESIAN_POINT('Ctrl Pts',(27.4293720419797,2.00385472437925,2.81527028497446));
#32672=CARTESIAN_POINT('Ctrl Pts',(27.5851582368823,-1.21809182407865,3.23377433657202));
#32673=CARTESIAN_POINT('Ctrl Pts',(27.7409444317848,-3.36326004332187,0.793614042292933));
#32674=CARTESIAN_POINT('Ctrl Pts',(27.8967306266874,-2.53517258006187,-2.34821560648262));
#32675=CARTESIAN_POINT('Ctrl Pts',(28.05251682159,0.533910506528028,-3.41398309224154));
#32676=CARTESIAN_POINT('Ctrl Pts',(28.2083030164925,3.13128822138237,-1.46211477286968));
#32677=CARTESIAN_POINT('Ctrl Pts',(28.3640892113951,2.9599971700504,1.7830513594197));
#32678=CARTESIAN_POINT('Ctrl Pts',(28.5198754062977,0.173103144446328,3.45046746880424));
#32679=CARTESIAN_POINT('Ctrl Pts',(28.6756616012002,-2.76896375813125,2.07058134389101));
#32680=CARTESIAN_POINT('Ctrl Pts',(28.8314477961028,-3.2589237700621,-1.14584557747595));
#32681=CARTESIAN_POINT('Ctrl Pts',(28.9353052593712,-1.671063172602,-2.60467617180897));
#32682=CARTESIAN_POINT('Ctrl Pts',(28.9872339910054,-0.742202251237312,
-2.84684032187586));
#32683=CARTESIAN_POINT('Ctrl Pts',(27.7778238829104,-2.9419205159921,0.00243417433800859));
#32684=CARTESIAN_POINT('Ctrl Pts',(27.8174594641694,-2.93560995158384,-0.730117559058909));
#32685=CARTESIAN_POINT('Ctrl Pts',(27.8570950454284,-2.65743809824621,-1.46695063553356));
#32686=CARTESIAN_POINT('Ctrl Pts',(27.8967306266874,-2.16167330950689,-2.00220524597985));
#32687=CARTESIAN_POINT('Ctrl Pts',(27.9486593583216,-1.5121448845319,-2.70347143506892));
#32688=CARTESIAN_POINT('Ctrl Pts',(28.0005880899558,-0.48911718900194,-3.05872726365523));
#32689=CARTESIAN_POINT('Ctrl Pts',(28.05251682159,0.455292944572102,-2.91104379138641));
#32690=CARTESIAN_POINT('Ctrl Pts',(28.1044455532242,1.39970307814614,-2.76336031911758));
#32691=CARTESIAN_POINT('Ctrl Pts',(28.1563742848584,2.26549564976426,-2.11273754599363));
#32692=CARTESIAN_POINT('Ctrl Pts',(28.2083030164925,2.66984342701799,-1.24656513738343));
#32693=CARTESIAN_POINT('Ctrl Pts',(28.2602317481267,3.07419120427171,-0.380392728773223));
#32694=CARTESIAN_POINT('Ctrl Pts',(28.3121604797609,3.01709418716105,0.701329315323246));
#32695=CARTESIAN_POINT('Ctrl Pts',(28.3640892113951,2.52406334100505,1.5200930222689));
#32696=CARTESIAN_POINT('Ctrl Pts',(28.4160179430293,2.03103249484904,2.33885672921455));
#32697=CARTESIAN_POINT('Ctrl Pts',(28.4679466746635,1.10206781964769,2.8946620990094));
#32698=CARTESIAN_POINT('Ctrl Pts',(28.5198754062977,0.147240998284077,2.94258376308795));
#32699=CARTESIAN_POINT('Ctrl Pts',(28.5659169375318,-0.699336369109807,
2.9850725111091));
#32700=CARTESIAN_POINT('Ctrl Pts',(28.6119584687659,-1.56624426411344,2.62830809441497));
#32701=CARTESIAN_POINT('Ctrl Pts',(28.658,-2.15060832247059,2.01293848078683));
#32702=CARTESIAN_POINT('',(22.6,-1.37977421736433,-1.93274596409627));
#32703=CARTESIAN_POINT('Ctrl Pts',(22.6,-1.3797742173643,-1.93274596409629));
#32704=CARTESIAN_POINT('Ctrl Pts',(22.6,-1.45785915848248,-1.89042312518908));
#32705=CARTESIAN_POINT('Ctrl Pts',(22.6,-1.53322062452788,-1.84365292533674));
#32706=CARTESIAN_POINT('Ctrl Pts',(22.6,-1.60541924836714,-1.7925389776215));
#32707=CARTESIAN_POINT('Ctrl Pts',(22.6,-1.67241398187154,-1.74510919124269));
#32708=CARTESIAN_POINT('Ctrl Pts',(22.6,-1.7366866559494,-1.6939390139514));
#32709=CARTESIAN_POINT('Ctrl Pts',(22.6,-1.79815525154635,-1.63938025328375));
#32710=CARTESIAN_POINT('Ctrl Pts',(22.6,-1.82774669609185,-1.61311525527802));
#32711=CARTESIAN_POINT('Ctrl Pts',(22.6,-1.85668798139578,-1.58606421212228));
#32712=CARTESIAN_POINT('Ctrl Pts',(22.6,-1.88496801744573,-1.55826263172972));
#32713=CARTESIAN_POINT('Ctrl Pts',(22.6,-1.89694635740944,-1.54648694725456));
#32714=CARTESIAN_POINT('Ctrl Pts',(22.6,-1.90880042781439,-1.5345820572415));
#32715=CARTESIAN_POINT('Ctrl Pts',(22.6,-1.92052581822529,-1.52255500426732));
#32716=CARTESIAN_POINT('Ctrl Pts',(22.6,-1.98100733369979,-1.46051746307855));
#32717=CARTESIAN_POINT('Ctrl Pts',(22.6,-2.03809982501458,-1.39520173965758));
#32718=CARTESIAN_POINT('Ctrl Pts',(22.6,-2.09171700828083,-1.32701838041071));
#32719=CARTESIAN_POINT('Ctrl Pts',(22.6,-2.1386320436388,-1.2673579410697));
#32720=CARTESIAN_POINT('Ctrl Pts',(22.6,-2.18288620426214,-1.20550076877931));
#32721=CARTESIAN_POINT('Ctrl Pts',(22.6,-2.2244039533604,-1.14169175518862));
#32722=CARTESIAN_POINT('Ctrl Pts',(22.6,-2.23783832694396,-1.12104434184867));
#32723=CARTESIAN_POINT('Ctrl Pts',(22.6,-2.25098603704135,-1.10019236804426));
#32724=CARTESIAN_POINT('Ctrl Pts',(22.6,-2.26384407676917,-1.07914361174352));
#32725=CARTESIAN_POINT('Ctrl Pts',(22.6,-2.27218773624139,-1.06548494692332));
#32726=CARTESIAN_POINT('Ctrl Pts',(22.6,-2.28040941692772,-1.05174341628636));
#32727=CARTESIAN_POINT('Ctrl Pts',(22.6,-2.28850824287345,-1.03792109526511));
#32728=CARTESIAN_POINT('Ctrl Pts',(22.6,-2.29616515491831,-1.02485299168755));
#32729=CARTESIAN_POINT('Ctrl Pts',(22.6,-2.30370706889497,-1.01172150964882));
#32730=CARTESIAN_POINT('Ctrl Pts',(22.6,-2.31113313207215,-0.998529628944857));
#32731=CARTESIAN_POINT('Ctrl Pts',(22.6,-2.35454850211762,-0.921405267261768));
#32732=CARTESIAN_POINT('Ctrl Pts',(22.6,-2.39401201422954,-0.842210569585459));
#32733=CARTESIAN_POINT('Ctrl Pts',(22.6,-2.42943733388716,-0.761342915874085));
#32734=CARTESIAN_POINT('Ctrl Pts',(22.6,-2.4654696596441,-0.679089610331911));
#32735=CARTESIAN_POINT('Ctrl Pts',(22.6,-2.49732484174602,-0.595104806954469));
#32736=CARTESIAN_POINT('Ctrl Pts',(22.6,-2.52487773536222,-0.509765448181997));
#32737=CARTESIAN_POINT('Ctrl Pts',(22.6,-2.5477911896283,-0.438795788095903));
#32738=CARTESIAN_POINT('Ctrl Pts',(22.6,-2.56772877983649,-0.366888349531481));
#32739=CARTESIAN_POINT('Ctrl Pts',(22.6,-2.584596243196,-0.29424448490606));
#32740=CARTESIAN_POINT('Ctrl Pts',(22.6,-2.59737320524494,-0.239217366623705));
#32741=CARTESIAN_POINT('Ctrl Pts',(22.6,-2.60838815722427,-0.183767373190182));
#32742=CARTESIAN_POINT('Ctrl Pts',(22.6,-2.61759113070643,-0.127978661306516));
#32743=CARTESIAN_POINT('Ctrl Pts',(22.6,-2.62055993379334,-0.10998168452769));
#32744=CARTESIAN_POINT('Ctrl Pts',(22.6,-2.62334060149709,-0.0919452294264881));
#32745=CARTESIAN_POINT('Ctrl Pts',(22.6,-2.62592758353743,-0.0739000925197149));
#32746=CARTESIAN_POINT('Ctrl Pts',(22.6,-2.63907517339903,0.0178091096886118));
#32747=CARTESIAN_POINT('Ctrl Pts',(22.6,-2.6472471121531,0.109869403253201));
#32748=CARTESIAN_POINT('Ctrl Pts',(22.6,-2.65032406207316,0.201881873939519));
#32749=CARTESIAN_POINT('Ctrl Pts',(22.6,-2.65219778541207,0.257913307104163));
#32750=CARTESIAN_POINT('Ctrl Pts',(22.6,-2.65218137509575,0.31392768209111));
#32751=CARTESIAN_POINT('Ctrl Pts',(22.6,-2.65023961232845,0.369839531880199));
#32752=CARTESIAN_POINT('Ctrl Pts',(22.6,-2.64715170229902,0.458753978399962));
#32753=CARTESIAN_POINT('Ctrl Pts',(22.6,-2.63919767846306,0.547409055573125));
#32754=CARTESIAN_POINT('Ctrl Pts',(22.6,-2.62661803880194,0.635544464197247));
#32755=CARTESIAN_POINT('Ctrl Pts',(22.6,-2.61933835618759,0.686547340205912));
#32756=CARTESIAN_POINT('Ctrl Pts',(22.6,-2.61050866025619,0.737376353293362));
#32757=CARTESIAN_POINT('Ctrl Pts',(22.6,-2.60016776191173,0.787981456082562));
#32758=CARTESIAN_POINT('Ctrl Pts',(22.6,-2.59279172176412,0.824077475733204));
#32759=CARTESIAN_POINT('Ctrl Pts',(22.6,-2.58464669361773,0.860059579007281));
#32760=CARTESIAN_POINT('Ctrl Pts',(22.6,-2.57574507716278,0.89590945104691));
#32761=CARTESIAN_POINT('Ctrl Pts',(22.6,-2.57127738066237,0.913902401952185));
#32762=CARTESIAN_POINT('Ctrl Pts',(22.6,-2.56661787459572,0.93186607753393));
#32763=CARTESIAN_POINT('Ctrl Pts',(22.6,-2.56177566668955,0.949771012880901));
#32764=CARTESIAN_POINT('Ctrl Pts',(22.6,-2.53764385793422,1.03900271956145));
#32765=CARTESIAN_POINT('Ctrl Pts',(22.6,-2.50895036688515,1.1268980164437));
#32766=CARTESIAN_POINT('Ctrl Pts',(22.6,-2.47598817745618,1.21317777136431));
#32767=CARTESIAN_POINT('Ctrl Pts',(22.6,-2.44237927848392,1.30115031253083));
#32768=CARTESIAN_POINT('Ctrl Pts',(22.6,-2.40433237097439,1.38744407152828));
#32769=CARTESIAN_POINT('Ctrl Pts',(22.6,-2.36210248902159,1.47176631907844));
#32770=CARTESIAN_POINT('Ctrl Pts',(22.6,-2.31948372457195,1.55686506527479));
#32771=CARTESIAN_POINT('Ctrl Pts',(22.6,-2.27260430302385,1.63995668918587));
#32772=CARTESIAN_POINT('Ctrl Pts',(22.6,-2.22167394745056,1.72073099208815));
#32773=CARTESIAN_POINT('Ctrl Pts',(22.6,-2.19223469061933,1.76742093606628));
#32774=CARTESIAN_POINT('Ctrl Pts',(22.6,-2.16144099506218,1.81333638138652));
#32775=CARTESIAN_POINT('Ctrl Pts',(22.6,-2.12932608668005,1.85841425069895));
#32776=CARTESIAN_POINT('Ctrl Pts',(22.6,-2.12079367180918,1.8703907158936));
#32777=CARTESIAN_POINT('Ctrl Pts',(22.6,-2.11216640274186,1.88231016366305));
#32778=CARTESIAN_POINT('Ctrl Pts',(22.6,-2.10344999573137,1.89416438598333));
#32779=CARTESIAN_POINT('Ctrl Pts',(22.6,-2.04526246313966,1.97329882139703));
#32780=CARTESIAN_POINT('Ctrl Pts',(22.6,-1.98324704259764,2.04933980788021));
#32781=CARTESIAN_POINT('Ctrl Pts',(22.6,-1.91768170146715,2.12198257731611));
#32782=CARTESIAN_POINT('Ctrl Pts',(22.6,-1.85187599989106,2.19489165282361));
#32783=CARTESIAN_POINT('Ctrl Pts',(22.6,-1.78249390688884,2.26437844634467));
#32784=CARTESIAN_POINT('Ctrl Pts',(22.6,-1.70976591886189,2.33011999619848));
#32785=CARTESIAN_POINT('Ctrl Pts',(22.6,-1.6383437830326,2.39468113738593));
#32786=CARTESIAN_POINT('Ctrl Pts',(22.6,-1.56369429611566,2.4556310976278));
#32787=CARTESIAN_POINT('Ctrl Pts',(22.6,-1.48599424012912,2.51263744458325));
#32788=CARTESIAN_POINT('Ctrl Pts',(22.6,-1.42232605236629,2.55934900425396));
#32789=CARTESIAN_POINT('Ctrl Pts',(22.6,-1.35660875961811,2.60341242494992));
#32790=CARTESIAN_POINT('Ctrl Pts',(22.6,-1.2889218540532,2.64462557919719));
#32791=CARTESIAN_POINT('Ctrl Pts',(22.6,-1.37977421736433,-1.93274596409627));
#32792=CARTESIAN_POINT('Ctrl Pts',(22.6460415312341,-0.820114607772339,
-2.32621799111725));
#32793=CARTESIAN_POINT('Ctrl Pts',(22.7440117941024,0.758470214248948,-2.63300441946709));
#32794=CARTESIAN_POINT('Ctrl Pts',(22.8939107886049,2.62282735660906,-0.938746401795666));
#32795=CARTESIAN_POINT('Ctrl Pts',(23.0496969835074,2.24240074214882,1.65328021767869));
#32796=CARTESIAN_POINT('Ctrl Pts',(23.2054831784101,-0.120664916242889,
2.78308709983206));
#32797=CARTESIAN_POINT('Ctrl Pts',(23.3384474812092,-2.04637284554299,1.64780428239185));
#32798=CARTESIAN_POINT('Ctrl Pts',(23.4194830523742,-2.36721675552049,0.4345208105624));
#32799=CARTESIAN_POINT('Ctrl Pts',(23.448589891905,-2.36840991602323,-0.000688909241090621));
#32800=CARTESIAN_POINT('Origin',(20.751410108095,0.,0.));
#32801=CARTESIAN_POINT('',(22.6,1.37702479013099,-1.93106208855767));
#32802=CARTESIAN_POINT('Origin',(22.6,0.,0.));
#32803=CARTESIAN_POINT('Ctrl Pts',(22.6,1.37702479013099,-1.93106208855767));
#32804=CARTESIAN_POINT('Ctrl Pts',(22.6519287316342,2.00708756429044,-1.48176940941637));
#32805=CARTESIAN_POINT('Ctrl Pts',(22.7557861949026,2.78394698441521,0.0732939610565424));
#32806=CARTESIAN_POINT('Ctrl Pts',(22.9115723898052,1.49072073679854,2.35522227267116));
#32807=CARTESIAN_POINT('Ctrl Pts',(23.0673585847077,-1.12180215515894,2.54924688068182));
#32808=CARTESIAN_POINT('Ctrl Pts',(23.1806378241377,-2.29982848865418,1.05373094085366));
#32809=CARTESIAN_POINT('Ctrl Pts',(23.2419883319334,-2.37405316087506,0.142149343728729));
#32810=CARTESIAN_POINT('Ctrl Pts',(23.251410108095,-2.37286196769524,0.00195470876282933));
#32811=CARTESIAN_POINT('Ctrl Pts',(22.2707660089946,1.70810875200394,-2.39535560853238));
#32812=CARTESIAN_POINT('Ctrl Pts',(22.3226947406288,2.48966021466954,-1.83803756825254));
#32813=CARTESIAN_POINT('Ctrl Pts',(22.4265522038972,3.45330326895732,0.0909163417005736));
#32814=CARTESIAN_POINT('Ctrl Pts',(22.5823383987997,1.84914110157534,2.92149844047583));
#32815=CARTESIAN_POINT('Ctrl Pts',(22.7381245937023,-1.39152184693901,3.16217321512214));
#32816=CARTESIAN_POINT('Ctrl Pts',(22.8939107886049,-3.40111157958131,0.61097941560448));
#32817=CARTESIAN_POINT('Ctrl Pts',(23.0496969835074,-2.40453763108011,-2.4821247976462));
#32818=CARTESIAN_POINT('Ctrl Pts',(23.20548317841,0.717935917613371,-3.38007436426549));
#32819=CARTESIAN_POINT('Ctrl Pts',(23.3612693733126,3.20561661195163,-1.29044022490378));
#32820=CARTESIAN_POINT('Ctrl Pts',(23.5170555682152,2.85953730127257,1.94020224751747));
#32821=CARTESIAN_POINT('Ctrl Pts',(23.6728417631178,-0.0144571353508022,
3.45555077544684));
#32822=CARTESIAN_POINT('Ctrl Pts',(23.8286279580203,-2.87565481901962,1.91619064272704));
#32823=CARTESIAN_POINT('Ctrl Pts',(23.9844141529229,-3.19472973788386,-1.31714785559497));
#32824=CARTESIAN_POINT('Ctrl Pts',(24.1402003478254,-0.68960129470691,-3.38608793893899));
#32825=CARTESIAN_POINT('Ctrl Pts',(24.295986542728,2.42514506376899,-2.46167280242748));
#32826=CARTESIAN_POINT('Ctrl Pts',(24.4517727376306,3.39602022813617,0.638909893803412));
#32827=CARTESIAN_POINT('Ctrl Pts',(24.6075589325332,1.36475126187535,3.1746825598677));
#32828=CARTESIAN_POINT('Ctrl Pts',(24.7633451274357,-1.8729823282135,2.90397922983507));
#32829=CARTESIAN_POINT('Ctrl Pts',(24.9191313223383,-3.45496565954171,0.066104969237162));
#32830=CARTESIAN_POINT('Ctrl Pts',(25.0749175172409,-1.98269651417726,-2.83020700980001));
#32831=CARTESIAN_POINT('Ctrl Pts',(25.2307037121434,1.24231233299229,-3.22456472193239));
#32832=CARTESIAN_POINT('Ctrl Pts',(25.386489907046,3.36909452241581,-0.768348565760258));
#32833=CARTESIAN_POINT('Ctrl Pts',(25.5422761019486,2.51753595578361,2.36710163085886));
#32834=CARTESIAN_POINT('Ctrl Pts',(25.6980622968512,-0.559570150281514,
3.40999103012744));
#32835=CARTESIAN_POINT('Ctrl Pts',(25.8538484917537,-3.14200602880735,1.43838635303248));
#32836=CARTESIAN_POINT('Ctrl Pts',(26.0096346866563,-2.94685160234359,-1.80477788365644));
#32837=CARTESIAN_POINT('Ctrl Pts',(26.1654208815589,-0.146626626641186,
-3.45248588722292));
#32838=CARTESIAN_POINT('Ctrl Pts',(26.3212070764614,2.78321855442789,-2.04813325762921));
#32839=CARTESIAN_POINT('Ctrl Pts',(26.476993271364,3.25264875345603,1.16680560889585));
#32840=CARTESIAN_POINT('Ctrl Pts',(26.6327794662666,0.846676835470829,3.35026863144008));
#32841=CARTESIAN_POINT('Ctrl Pts',(26.7885656611691,-2.30776977335729,2.57203035539396));
#32842=CARTESIAN_POINT('Ctrl Pts',(26.9443518560717,-3.42211190186477,-0.479923642607166));
#32843=CARTESIAN_POINT('Ctrl Pts',(27.1001380509743,-1.51123330277005,-3.10762789310822));
#32844=CARTESIAN_POINT('Ctrl Pts',(27.2559242458769,1.73558010371673,-2.98811008398895));
#32845=CARTESIAN_POINT('Ctrl Pts',(27.4117104407794,3.44815415895054,-0.227093009036346));
#32846=CARTESIAN_POINT('Ctrl Pts',(27.567496635682,2.1124088583074,2.73476555708426));
#32847=CARTESIAN_POINT('Ctrl Pts',(27.7232828305846,-1.09057038322062,3.27887037392547));
#32848=CARTESIAN_POINT('Ctrl Pts',(27.8790690254871,-3.32980739272074,0.924731019136299));
#32849=CARTESIAN_POINT('Ctrl Pts',(28.0348552203897,-2.62476217261374,-2.24754963466227));
#32850=CARTESIAN_POINT('Ctrl Pts',(28.1906414152923,0.399298518841041,-3.4316516702305));
#32851=CARTESIAN_POINT('Ctrl Pts',(28.3464276101949,3.07298101041792,-1.5846967094207));
#32852=CARTESIAN_POINT('Ctrl Pts',(28.5022138050974,3.0248495908613,1.66848859787707));
#32853=CARTESIAN_POINT('Ctrl Pts',(28.6060712683658,1.21780515048259,2.84495003511031));
#32854=CARTESIAN_POINT('Ctrl Pts',(28.658,0.261701021631923,2.93033728012268));
#32855=CARTESIAN_POINT('Ctrl Pts',(22.3805106726631,1.59774743137962,-2.24059110187414));
#32856=CARTESIAN_POINT('Ctrl Pts',(22.4324394042973,2.32880266454317,-1.71928151530715));
#32857=CARTESIAN_POINT('Ctrl Pts',(22.5362968675656,3.23018450744328,0.0850422148192308));
#32858=CARTESIAN_POINT('Ctrl Pts',(22.6920830624682,1.72966764664974,2.73273971787427));
#32859=CARTESIAN_POINT('Ctrl Pts',(22.8478692573708,-1.30161528301232,2.95786443697537));
#32860=CARTESIAN_POINT('Ctrl Pts',(23.0036554522734,-3.18136493577254,0.571503887420878));
#32861=CARTESIAN_POINT('Ctrl Pts',(23.1594416471759,-2.24917987171874,-2.32175411264079));
#32862=CARTESIAN_POINT('Ctrl Pts',(23.3152278420785,0.671549903901719,-3.16168694003907));
#32863=CARTESIAN_POINT('Ctrl Pts',(23.471014036981,2.99850094540219,-1.20706456908558));
#32864=CARTESIAN_POINT('Ctrl Pts',(23.6268002318837,2.67478190289836,1.81484530987337));
#32865=CARTESIAN_POINT('Ctrl Pts',(23.7825864267862,-0.0135230563304296,
3.23228680199357));
#32866=CARTESIAN_POINT('Ctrl Pts',(23.9383726216888,-2.68985806391585,1.79238510069044));
#32867=CARTESIAN_POINT('Ctrl Pts',(24.0941588165913,-2.98831747490762,-1.23204661328215));
#32868=CARTESIAN_POINT('Ctrl Pts',(24.2499450114939,-0.645045987851415,
-3.16731197619483));
#32869=CARTESIAN_POINT('Ctrl Pts',(24.4057312063965,2.26845585318501,-2.30262352579206));
#32870=CARTESIAN_POINT('Ctrl Pts',(24.561517401299,3.17660253777874,0.597629770651206));
#32871=CARTESIAN_POINT('Ctrl Pts',(24.7173035962016,1.27657435194057,2.96956554992383));
#32872=CARTESIAN_POINT('Ctrl Pts',(24.8730897911042,-1.75196848585414,2.71635242768082));
#32873=CARTESIAN_POINT('Ctrl Pts',(25.0288759860068,-3.23173949056894,0.0618339111465752));
#32874=CARTESIAN_POINT('Ctrl Pts',(25.1846621809093,-1.85459401166088,-2.64734664866943));
#32875=CARTESIAN_POINT('Ctrl Pts',(25.3404483758119,1.16204623193985,-3.01622481340282));
#32876=CARTESIAN_POINT('Ctrl Pts',(25.4962345707145,3.15141650843352,-0.718705378628512));
#32877=CARTESIAN_POINT('Ctrl Pts',(25.6520207656171,2.35487734726496,2.21416262054873));
#32878=CARTESIAN_POINT('Ctrl Pts',(25.8078069605196,-0.523416187195402,
3.18967068286592));
#32879=CARTESIAN_POINT('Ctrl Pts',(25.9635931554222,-2.93900025745823,1.34545186200406));
#32880=CARTESIAN_POINT('Ctrl Pts',(26.1193793503248,-2.75645480580648,-1.68817074699713));
#32881=CARTESIAN_POINT('Ctrl Pts',(26.2751655452273,-0.137153044742009,
-3.22941993694093));
#32882=CARTESIAN_POINT('Ctrl Pts',(26.4309517401299,2.60339412879199,-1.91580287125224));
#32883=CARTESIAN_POINT('Ctrl Pts',(26.5867379350325,3.04249432884032,1.09141801559505));
#32884=CARTESIAN_POINT('Ctrl Pts',(26.7425241299351,0.791972839841186,3.13380696283837));
#32885=CARTESIAN_POINT('Ctrl Pts',(26.8983103248376,-2.15866420874626,2.40585085050347));
#32886=CARTESIAN_POINT('Ctrl Pts',(27.0540965197402,-3.20100842214141,-0.448915659693424));
#32887=CARTESIAN_POINT('Ctrl Pts',(27.2098827146427,-1.41359215265622,-2.90684330144212));
#32888=CARTESIAN_POINT('Ctrl Pts',(27.3656689095453,1.6234438523974,-2.79504756694899));
#32889=CARTESIAN_POINT('Ctrl Pts',(27.5214551044479,3.22536808268251,-0.212420474660298));
#32890=CARTESIAN_POINT('Ctrl Pts',(27.6772412993505,1.97592560978601,2.5580716913549));
#32891=CARTESIAN_POINT('Ctrl Pts',(27.833027494253,-1.0201083663351,3.06702176405338));
#32892=CARTESIAN_POINT('Ctrl Pts',(27.9888136891556,-3.11466772971383,0.864983923774584));
#32893=CARTESIAN_POINT('Ctrl Pts',(28.1445998840582,-2.45517565222704,-2.10233490781362));
#32894=CARTESIAN_POINT('Ctrl Pts',(28.3003860789607,0.373499744722629,-3.20993182375997));
#32895=CARTESIAN_POINT('Ctrl Pts',(28.4561722738633,2.87443496224312,-1.48230907079083));
#32896=CARTESIAN_POINT('Ctrl Pts',(28.6119584687659,2.82941332537425,1.56068714501741));
#32897=CARTESIAN_POINT('Ctrl Pts',(28.7158159320343,1.13912246443424,2.66113712353977));
#32898=CARTESIAN_POINT('Ctrl Pts',(28.7677446636685,0.244792455170829,2.74100747794843));
#32899=CARTESIAN_POINT('Ctrl Pts',(22.4902553363315,1.4873861107553,-2.08582659521591));
#32900=CARTESIAN_POINT('Ctrl Pts',(22.5421840679657,2.16794511441681,-1.60052546236176));
#32901=CARTESIAN_POINT('Ctrl Pts',(22.6460415312341,3.00706574592924,0.0791680879378876));
#32902=CARTESIAN_POINT('Ctrl Pts',(22.8018277261367,1.61019419172414,2.54398099527271));
#32903=CARTESIAN_POINT('Ctrl Pts',(22.9576139210392,-1.21170871908563,2.7535556588286));
#32904=CARTESIAN_POINT('Ctrl Pts',(23.1134001159418,-2.96161829196376,0.532028359237276));
#32905=CARTESIAN_POINT('Ctrl Pts',(23.2691863108444,-2.09382211235737,-2.16138342763538));
#32906=CARTESIAN_POINT('Ctrl Pts',(23.4249725057469,0.625163890190072,-2.94329951581265));
#32907=CARTESIAN_POINT('Ctrl Pts',(23.5807587006496,2.79138527885274,-1.12368891326739));
#32908=CARTESIAN_POINT('Ctrl Pts',(23.7365448955521,2.49002650452417,1.68948837222927));
#32909=CARTESIAN_POINT('Ctrl Pts',(23.8923310904547,-0.0125889773100609,
3.0090228285403));
#32910=CARTESIAN_POINT('Ctrl Pts',(24.0481172853572,-2.50406130881207,1.66857955865383));
#32911=CARTESIAN_POINT('Ctrl Pts',(24.2039034802599,-2.78190521193138,-1.14694537096932));
#32912=CARTESIAN_POINT('Ctrl Pts',(24.3596896751623,-0.600490680995917,
-2.94853601345067));
#32913=CARTESIAN_POINT('Ctrl Pts',(24.515475870065,2.11176664260102,-2.14357424915663));
#32914=CARTESIAN_POINT('Ctrl Pts',(24.6712620649675,2.95718484742131,0.556349647498999));
#32915=CARTESIAN_POINT('Ctrl Pts',(24.8270482598701,1.18839744200578,2.76444853997997));
#32916=CARTESIAN_POINT('Ctrl Pts',(24.9828344547727,-1.63095464349477,2.52872562552656));
#32917=CARTESIAN_POINT('Ctrl Pts',(25.1386206496752,-3.00851332159618,0.0575628530559896));
#32918=CARTESIAN_POINT('Ctrl Pts',(25.2944068445778,-1.7264915091445,-2.46448628753886));
#32919=CARTESIAN_POINT('Ctrl Pts',(25.4501930394804,1.08178013088741,-2.80788490487326));
#32920=CARTESIAN_POINT('Ctrl Pts',(25.6059792343829,2.93373849445125,-0.669062191496764));
#32921=CARTESIAN_POINT('Ctrl Pts',(25.7617654292855,2.19221873874631,2.06122361023859));
#32922=CARTESIAN_POINT('Ctrl Pts',(25.9175516241881,-0.48726222410929,2.9693503356044));
#32923=CARTESIAN_POINT('Ctrl Pts',(26.0733378190906,-2.7359944861091,1.25251737097565));
#32924=CARTESIAN_POINT('Ctrl Pts',(26.2291240139933,-2.56605800926939,-1.57156361033782));
#32925=CARTESIAN_POINT('Ctrl Pts',(26.3849102088958,-0.127679462842828,
-3.00635398665893));
#32926=CARTESIAN_POINT('Ctrl Pts',(26.5406964037984,2.42356970315608,-1.78347248487528));
#32927=CARTESIAN_POINT('Ctrl Pts',(26.6964825987009,2.8323399042246,1.01603042229426));
#32928=CARTESIAN_POINT('Ctrl Pts',(26.8522687936035,0.737268844211538,2.91734529423666));
#32929=CARTESIAN_POINT('Ctrl Pts',(27.0080549885061,-2.00955864413522,2.23967134561299));
#32930=CARTESIAN_POINT('Ctrl Pts',(27.1638411834087,-2.97990494241805,-0.417907676779675));
#32931=CARTESIAN_POINT('Ctrl Pts',(27.3196273783112,-1.3159510025424,-2.70605870977603));
#32932=CARTESIAN_POINT('Ctrl Pts',(27.4754135732138,1.51130760107806,-2.60198504990902));
#32933=CARTESIAN_POINT('Ctrl Pts',(27.6311997681163,3.0025820064145,-0.197747940284252));
#32934=CARTESIAN_POINT('Ctrl Pts',(27.7869859630189,1.83944236126462,2.38137782562555));
#32935=CARTESIAN_POINT('Ctrl Pts',(27.9427721579215,-0.949646349449587,
2.8551731541813));
#32936=CARTESIAN_POINT('Ctrl Pts',(28.0985583528241,-2.89952806670692,0.805236828412871));
#32937=CARTESIAN_POINT('Ctrl Pts',(28.2543445477266,-2.28558913184034,-1.95712018096498));
#32938=CARTESIAN_POINT('Ctrl Pts',(28.4101307426292,0.347700970604219,-2.98821197728943));
#32939=CARTESIAN_POINT('Ctrl Pts',(28.5659169375318,2.67588891406832,-1.37992143216097));
#32940=CARTESIAN_POINT('Ctrl Pts',(28.7217031324344,2.6339770598872,1.45288569215775));
#32941=CARTESIAN_POINT('Ctrl Pts',(28.8255605957027,1.06043977838589,2.47732421196922));
#32942=CARTESIAN_POINT('Ctrl Pts',(28.8774893273369,0.227883888709735,2.55167767577418));
#32943=CARTESIAN_POINT('Ctrl Pts',(22.6,1.37702479013099,-1.93106208855767));
#32944=CARTESIAN_POINT('Ctrl Pts',(22.6519287316342,2.00708756429044,-1.48176940941637));
#32945=CARTESIAN_POINT('Ctrl Pts',(22.7557861949026,2.78394698441521,0.0732939610565424));
#32946=CARTESIAN_POINT('Ctrl Pts',(22.9115723898052,1.49072073679854,2.35522227267116));
#32947=CARTESIAN_POINT('Ctrl Pts',(23.0673585847077,-1.12180215515894,2.54924688068182));
#32948=CARTESIAN_POINT('Ctrl Pts',(23.2231447796103,-2.74187164815499,0.492552831053676));
#32949=CARTESIAN_POINT('Ctrl Pts',(23.3789309745128,-1.938464352996,-2.00101274262997));
#32950=CARTESIAN_POINT('Ctrl Pts',(23.5347171694154,0.578777876478422,-2.72491209158622));
#32951=CARTESIAN_POINT('Ctrl Pts',(23.690503364318,2.58426961230329,-1.04031325744919));
#32952=CARTESIAN_POINT('Ctrl Pts',(23.8462895592206,2.30527110614996,1.56413143458517));
#32953=CARTESIAN_POINT('Ctrl Pts',(24.0020757541231,-0.0116548982896913,
2.78575885508703));
#32954=CARTESIAN_POINT('Ctrl Pts',(24.1578619490257,-2.3182645537083,1.54477401661722));
#32955=CARTESIAN_POINT('Ctrl Pts',(24.3136481439283,-2.57549294895514,-1.06184412865649));
#32956=CARTESIAN_POINT('Ctrl Pts',(24.4694343388309,-0.555935374140417,
-2.72976005070651));
#32957=CARTESIAN_POINT('Ctrl Pts',(24.6252205337334,1.95507743201704,-1.9845249725212));
#32958=CARTESIAN_POINT('Ctrl Pts',(24.781006728636,2.73776715706389,0.51506952434679));
#32959=CARTESIAN_POINT('Ctrl Pts',(24.9367929235385,1.10022053207099,2.55933153003611));
#32960=CARTESIAN_POINT('Ctrl Pts',(25.0925791184411,-1.50994080113541,2.3410988233723));
#32961=CARTESIAN_POINT('Ctrl Pts',(25.2483653133437,-2.7852871526234,0.0532917949654058));
#32962=CARTESIAN_POINT('Ctrl Pts',(25.4041515082462,-1.59838900662812,-2.28162592640829));
#32963=CARTESIAN_POINT('Ctrl Pts',(25.5599377031489,1.00151402983497,-2.59954499634369));
#32964=CARTESIAN_POINT('Ctrl Pts',(25.7157238980514,2.71606048046896,-0.619419004365017));
#32965=CARTESIAN_POINT('Ctrl Pts',(25.871510092954,2.02956013022766,1.90828459992846));
#32966=CARTESIAN_POINT('Ctrl Pts',(26.0272962878565,-0.451108261023179,
2.74902998834288));
#32967=CARTESIAN_POINT('Ctrl Pts',(26.1830824827591,-2.53298871475997,1.15958287994724));
#32968=CARTESIAN_POINT('Ctrl Pts',(26.3388686776617,-2.37566121273229,-1.45495647367851));
#32969=CARTESIAN_POINT('Ctrl Pts',(26.4946548725642,-0.118205880943649,
-2.78328803637694));
#32970=CARTESIAN_POINT('Ctrl Pts',(26.6504410674669,2.24374527752018,-1.65114209849832));
#32971=CARTESIAN_POINT('Ctrl Pts',(26.8062272623694,2.62218547960889,0.940642828993458));
#32972=CARTESIAN_POINT('Ctrl Pts',(26.962013457272,0.682564848581893,2.70088362563495));
#32973=CARTESIAN_POINT('Ctrl Pts',(27.1177996521745,-1.86045307952419,2.07349184072251));
#32974=CARTESIAN_POINT('Ctrl Pts',(27.2735858470771,-2.75880146269469,-0.386899693865931));
#32975=CARTESIAN_POINT('Ctrl Pts',(27.4293720419797,-1.21830985242857,-2.50527411810993));
#32976=CARTESIAN_POINT('Ctrl Pts',(27.5851582368822,1.39917134975873,-2.40892253286906));
#32977=CARTESIAN_POINT('Ctrl Pts',(27.7409444317848,2.77979593014647,-0.183075405908203));
#32978=CARTESIAN_POINT('Ctrl Pts',(27.8967306266874,1.70295911274323,2.20468395989619));
#32979=CARTESIAN_POINT('Ctrl Pts',(28.05251682159,-0.879184332564077,2.64332454430922));
#32980=CARTESIAN_POINT('Ctrl Pts',(28.2083030164925,-2.6843884037,0.745489733051156));
#32981=CARTESIAN_POINT('Ctrl Pts',(28.3640892113951,-2.11600261145364,-1.81190545411633));
#32982=CARTESIAN_POINT('Ctrl Pts',(28.5198754062977,0.321902196485808,-2.7664921308189));
#32983=CARTESIAN_POINT('Ctrl Pts',(28.6756616012002,2.47734286589352,-1.27753379353111));
#32984=CARTESIAN_POINT('Ctrl Pts',(28.8314477961028,2.43854079440016,1.34508423929808));
#32985=CARTESIAN_POINT('Ctrl Pts',(28.9353052593712,0.981757092337547,2.29351130039867));
#32986=CARTESIAN_POINT('Ctrl Pts',(28.9872339910054,0.210975322248641,2.36234787359992));
#32987=CARTESIAN_POINT('Ctrl Pts',(22.6,1.29193968544099,2.64724960214528));
#32988=CARTESIAN_POINT('Ctrl Pts',(22.6,1.37398662210897,2.59799179582031));
#32989=CARTESIAN_POINT('Ctrl Pts',(22.6,1.45331123519463,2.54465519870452));
#32990=CARTESIAN_POINT('Ctrl Pts',(22.6,1.52954787739396,2.48723802283488));
#32991=CARTESIAN_POINT('Ctrl Pts',(22.6,1.53975420128136,2.4795511904047));
#32992=CARTESIAN_POINT('Ctrl Pts',(22.6,1.54990512670829,2.471791166031));
#32993=CARTESIAN_POINT('Ctrl Pts',(22.6,1.55999972524662,2.46395789450524));
#32994=CARTESIAN_POINT('Ctrl Pts',(22.6,1.63744923949508,2.4038581221029));
#32995=CARTESIAN_POINT('Ctrl Pts',(22.6,1.71158671352519,2.33944889993133));
#32996=CARTESIAN_POINT('Ctrl Pts',(22.6,1.7822309969812,2.27110880309472));
#32997=CARTESIAN_POINT('Ctrl Pts',(22.6,1.80301535614779,2.25100236208289));
#32998=CARTESIAN_POINT('Ctrl Pts',(22.6,1.82349704371371,2.23055549420075));
#32999=CARTESIAN_POINT('Ctrl Pts',(22.6,1.84367067623173,2.20977747618807));
#33000=CARTESIAN_POINT('Ctrl Pts',(22.6,1.85694131862264,2.19610925622859));
#33001=CARTESIAN_POINT('Ctrl Pts',(22.6,1.87007864940316,2.18229773526248));
#33002=CARTESIAN_POINT('Ctrl Pts',(22.6,1.88308104907989,2.16834552726226));
#33003=CARTESIAN_POINT('Ctrl Pts',(22.6,1.89645232297084,2.15399749926799));
#33004=CARTESIAN_POINT('Ctrl Pts',(22.6,1.90967535655003,2.13950656026653));
#33005=CARTESIAN_POINT('Ctrl Pts',(22.6,1.92274364758183,2.12488175434569));
#33006=CARTESIAN_POINT('Ctrl Pts',(22.6,1.98743002993418,2.0524908208011));
#33007=CARTESIAN_POINT('Ctrl Pts',(22.6,2.04837002339202,1.97677788797286));
#33008=CARTESIAN_POINT('Ctrl Pts',(22.6,2.10540137231736,1.89812284077031));
#33009=CARTESIAN_POINT('Ctrl Pts',(22.6,2.15306292861443,1.83239018617011));
#33010=CARTESIAN_POINT('Ctrl Pts',(22.6,2.19799397733902,1.76460187700287));
#33011=CARTESIAN_POINT('Ctrl Pts',(22.6,2.24007370157356,1.69496974001289));
#33012=CARTESIAN_POINT('Ctrl Pts',(22.6,2.2588040734674,1.66397533961436));
#33013=CARTESIAN_POINT('Ctrl Pts',(22.6,2.27696918818612,1.63261554623335));
#33014=CARTESIAN_POINT('Ctrl Pts',(22.6,2.2945567623349,1.60090880756888));
#33015=CARTESIAN_POINT('Ctrl Pts',(22.6,2.30328860155935,1.58516711732737));
#33016=CARTESIAN_POINT('Ctrl Pts',(22.6,2.31187806677236,1.56933990751256));
#33017=CARTESIAN_POINT('Ctrl Pts',(22.6,2.32032355901159,1.55342943411423));
#33018=CARTESIAN_POINT('Ctrl Pts',(22.6,2.32804618004994,1.53888077867587));
#33019=CARTESIAN_POINT('Ctrl Pts',(22.6,2.33564454313757,1.52426973302578));
#33020=CARTESIAN_POINT('Ctrl Pts',(22.6,2.34311514756603,1.50960353912746));
#33021=CARTESIAN_POINT('Ctrl Pts',(22.6,2.3862343690969,1.42495244164634));
#33022=CARTESIAN_POINT('Ctrl Pts',(22.6,2.42513144916236,1.33840899559929));
#33023=CARTESIAN_POINT('Ctrl Pts',(22.6,2.45965235719831,1.25032466278114));
#33024=CARTESIAN_POINT('Ctrl Pts',(22.6,2.49387162064543,1.16301001314535));
#33025=CARTESIAN_POINT('Ctrl Pts',(22.6,2.52379105451494,1.07418035409301));
#33026=CARTESIAN_POINT('Ctrl Pts',(22.6,2.54921046539056,0.98416944937067));
#33027=CARTESIAN_POINT('Ctrl Pts',(22.6,2.57014848001453,0.910027304668119));
#33028=CARTESIAN_POINT('Ctrl Pts',(22.6,2.58803245793096,0.83508332520754));
#33029=CARTESIAN_POINT('Ctrl Pts',(22.6,2.60272312322177,0.759526199301805));
#33030=CARTESIAN_POINT('Ctrl Pts',(22.6,2.61374112218987,0.702858354872504));
#33031=CARTESIAN_POINT('Ctrl Pts',(22.6,2.62296238253348,0.645845632245045));
#33032=CARTESIAN_POINT('Ctrl Pts',(22.6,2.63031846040409,0.588570176538994));
#33033=CARTESIAN_POINT('Ctrl Pts',(22.6,2.63217022162964,0.574152103495507));
#33034=CARTESIAN_POINT('Ctrl Pts',(22.6,2.63390374573031,0.559717395949854));
#33035=CARTESIAN_POINT('Ctrl Pts',(22.6,2.63551785486944,0.545267396301203));
#33036=CARTESIAN_POINT('Ctrl Pts',(22.6,2.63700943918069,0.531914276458778));
#33037=CARTESIAN_POINT('Ctrl Pts',(22.6,2.63839851735333,0.518552496504733));
#33038=CARTESIAN_POINT('Ctrl Pts',(22.6,2.63968370751675,0.505190950925346));
#33039=CARTESIAN_POINT('Ctrl Pts',(22.6,2.64822927439902,0.416346525680822));
#33040=CARTESIAN_POINT('Ctrl Pts',(22.6,2.65219771421662,0.327406838635517));
#33041=CARTESIAN_POINT('Ctrl Pts',(22.6,2.65141649101387,0.238668286707819));
#33042=CARTESIAN_POINT('Ctrl Pts',(22.6,2.65092714796485,0.183084180382702));
#33043=CARTESIAN_POINT('Ctrl Pts',(22.6,2.64857327480457,0.127578997259634));
#33044=CARTESIAN_POINT('Ctrl Pts',(22.6,2.6443021234377,0.0722273116339143));
#33045=CARTESIAN_POINT('Ctrl Pts',(22.6,2.63733327280372,-0.018085017836793));
#33046=CARTESIAN_POINT('Ctrl Pts',(22.6,2.6252624315387,-0.107990203752847));
#33047=CARTESIAN_POINT('Ctrl Pts',(22.6,2.60828201361834,-0.197151736827924));
#33048=CARTESIAN_POINT('Ctrl Pts',(22.6,2.59124313592887,-0.28662023305671));
#33049=CARTESIAN_POINT('Ctrl Pts',(22.6,2.56926019798414,-0.375340802433049));
#33050=CARTESIAN_POINT('Ctrl Pts',(22.6,2.54248600040002,-0.462941832765398));
#33051=CARTESIAN_POINT('Ctrl Pts',(22.6,2.53837999571101,-0.476376044572389));
#33052=CARTESIAN_POINT('Ctrl Pts',(22.6,2.53416363894075,-0.489775921708853));
#33053=CARTESIAN_POINT('Ctrl Pts',(22.6,2.5298392091435,-0.503136034212508));
#33054=CARTESIAN_POINT('Ctrl Pts',(22.6,2.50253277200761,-0.587497924522625));
#33055=CARTESIAN_POINT('Ctrl Pts',(22.6,2.47090442181699,-0.670330946599523));
#33056=CARTESIAN_POINT('Ctrl Pts',(22.6,2.43517017876197,-0.751334282795894));
#33057=CARTESIAN_POINT('Ctrl Pts',(22.6,2.39947016711518,-0.83226002232216));
#33058=CARTESIAN_POINT('Ctrl Pts',(22.6,2.35967146038532,-0.911360358667436));
#33059=CARTESIAN_POINT('Ctrl Pts',(22.6,2.31594727372697,-0.988305313713532));
#33060=CARTESIAN_POINT('Ctrl Pts',(22.6,2.2729032797118,-1.06405327925901));
#33061=CARTESIAN_POINT('Ctrl Pts',(22.6,2.22605430689985,-1.137713018672));
#33062=CARTESIAN_POINT('Ctrl Pts',(22.6,2.17553481696067,-1.20893040656016));
#33063=CARTESIAN_POINT('Ctrl Pts',(22.6,2.15829884607901,-1.23322797617905));
#33064=CARTESIAN_POINT('Ctrl Pts',(22.6,2.14063540467206,-1.25724087327014));
#33065=CARTESIAN_POINT('Ctrl Pts',(22.6,2.12254920670209,-1.28095377076072));
#33066=CARTESIAN_POINT('Ctrl Pts',(22.6,2.11108446021501,-1.29598525270375));
#33067=CARTESIAN_POINT('Ctrl Pts',(22.6,2.09944983480608,-1.3108961744379));
#33068=CARTESIAN_POINT('Ctrl Pts',(22.6,2.08764647715969,-1.32568248351855));
#33069=CARTESIAN_POINT('Ctrl Pts',(22.6,2.07921581304034,-1.33624374999529));
#33070=CARTESIAN_POINT('Ctrl Pts',(22.6,2.07070458118542,-1.34673450751064));
#33071=CARTESIAN_POINT('Ctrl Pts',(22.6,2.06211537646975,-1.35715132281721));
#33072=CARTESIAN_POINT('Ctrl Pts',(22.6,2.007856874164,-1.42295494678941));
#33073=CARTESIAN_POINT('Ctrl Pts',(22.6,1.95046520729726,-1.48584152571506));
#33074=CARTESIAN_POINT('Ctrl Pts',(22.6,1.89010219144091,-1.54551632835672));
#33075=CARTESIAN_POINT('Ctrl Pts',(22.6,1.83067278976528,-1.60426816117674));
#33076=CARTESIAN_POINT('Ctrl Pts',(22.6,1.76836259681773,-1.65990731572679));
#33077=CARTESIAN_POINT('Ctrl Pts',(22.6,1.70330015578668,-1.71211004597693));
#33078=CARTESIAN_POINT('Ctrl Pts',(22.6,1.64025601666085,-1.76269339539456));
#33079=CARTESIAN_POINT('Ctrl Pts',(22.6,1.57462716209707,-1.81005050265833));
#33080=CARTESIAN_POINT('Ctrl Pts',(22.6,1.50651496632111,-1.85384102298016));
#33081=CARTESIAN_POINT('Ctrl Pts',(22.6,1.46429839471039,-1.88098279422944));
#33082=CARTESIAN_POINT('Ctrl Pts',(22.6,1.42112754045947,-1.90675349235672));
#33083=CARTESIAN_POINT('Ctrl Pts',(22.6,1.37702479013099,-1.93106208855767));
#33084=CARTESIAN_POINT('Ctrl Pts',(28.658,0.261701021631923,2.93033728012268));
#33085=CARTESIAN_POINT('Ctrl Pts',(28.6060712683658,1.21780515048259,2.84495003511031));
#33086=CARTESIAN_POINT('Ctrl Pts',(28.5541425367316,2.12132737067194,2.25671931649369));
#33087=CARTESIAN_POINT('Ctrl Pts',(28.5022138050974,2.58111038402606,1.42040640596909));
#33088=CARTESIAN_POINT('Ctrl Pts',(28.4502850734632,3.04089339738017,0.584093495444484));
#33089=CARTESIAN_POINT('Ctrl Pts',(28.3983563418291,3.05693720389905,-0.500301606988106));
#33090=CARTESIAN_POINT('Ctrl Pts',(28.3464276101949,2.61934535856234,-1.35032498500603));
#33091=CARTESIAN_POINT('Ctrl Pts',(28.2944988785607,2.18175351322563,-2.20034836302396));
#33092=CARTESIAN_POINT('Ctrl Pts',(28.2425701469265,1.29052601603334,-2.81600001662723));
#33093=CARTESIAN_POINT('Ctrl Pts',(28.1906414152923,0.340902152194731,-2.9264755041675));
#33094=CARTESIAN_POINT('Ctrl Pts',(28.1387126836581,-0.608721711643891,
-3.03695099170776));
#33095=CARTESIAN_POINT('Ctrl Pts',(28.0867839520239,-1.61674194212883,-2.64225031318501));
#33096=CARTESIAN_POINT('Ctrl Pts',(28.0348552203897,-2.23825959405579,-1.91618653162386));
#33097=CARTESIAN_POINT('Ctrl Pts',(27.9972955192897,-2.68779911678517,-1.39102949896014));
#33098=CARTESIAN_POINT('Ctrl Pts',(27.9597358181896,-2.93513860722871,-0.692518823009792));
#33099=CARTESIAN_POINT('Ctrl Pts',(27.9221761170896,-2.94084529159276,0.00236346891266642));
#33100=CARTESIAN_POINT('Origin',(25.6,0.,0.));
#33101=CARTESIAN_POINT('Origin',(28.658,0.,0.));
#33102=CARTESIAN_POINT('Origin',(2.,4.6,0.));
#33103=CARTESIAN_POINT('',(2.,-4.6,-5.63337527607782E-16));
#33104=CARTESIAN_POINT('Origin',(2.,0.,0.));
#33105=CARTESIAN_POINT('Origin',(2.2,0.,0.));
#33106=CARTESIAN_POINT('',(2.4,-5.,-6.12323399573676E-16));
#33107=CARTESIAN_POINT('Origin',(2.4,0.,0.));
#33108=CARTESIAN_POINT('',(2.2,-4.8,-5.87830463590729E-16));
#33109=CARTESIAN_POINT('Origin',(12.5,0.,0.));
#33110=CARTESIAN_POINT('',(22.6,-5.,-6.12323399573677E-16));
#33111=CARTESIAN_POINT('Origin',(22.6,0.,0.));
#33112=CARTESIAN_POINT('',(12.5,-5.,-6.12323399573677E-16));
#33113=CARTESIAN_POINT('Origin',(22.6,3.,0.));
#33114=CARTESIAN_POINT('Origin',(28.8,0.,0.));
#33115=CARTESIAN_POINT('',(29.,-2.6,-3.18408167778312E-16));
#33116=CARTESIAN_POINT('Origin',(29.,0.,0.));
#33117=CARTESIAN_POINT('',(28.8,-2.8,-3.42901103761259E-16));
#33118=CARTESIAN_POINT('Origin',(29.,0.,0.));
#38505=UNCERTAINTY_MEASURE_WITH_UNIT(LENGTH_MEASURE(0.01),#38529,
'DISTANCE_ACCURACY_VALUE',
'Maximum model space distance between geometric entities at asserted c
onnectivities');
#38514=UNCERTAINTY_MEASURE_WITH_UNIT(LENGTH_MEASURE(0.01),#38529,
'DISTANCE_ACCURACY_VALUE',
'Maximum model space distance between geometric entities at asserted c
onnectivities');
#38519=(
GEOMETRIC_REPRESENTATION_CONTEXT(3)
GLOBAL_UNCERTAINTY_ASSIGNED_CONTEXT((#38505))
GLOBAL_UNIT_ASSIGNED_CONTEXT((#38529,#38531,#38532))
REPRESENTATION_CONTEXT('','3D')
);
#38528=(
GEOMETRIC_REPRESENTATION_CONTEXT(3)
GLOBAL_UNCERTAINTY_ASSIGNED_CONTEXT((#38514))
GLOBAL_UNIT_ASSIGNED_CONTEXT((#38529,#38531,#38532))
REPRESENTATION_CONTEXT('','3D')
);
#38529=(
LENGTH_UNIT()
NAMED_UNIT(*)
SI_UNIT(.MILLI.,.METRE.)
);
#38531=(
NAMED_UNIT(*)
PLANE_ANGLE_UNIT()
SI_UNIT($,.RADIAN.)
);
#38532=(
NAMED_UNIT(*)
SI_UNIT($,.STERADIAN.)
SOLID_ANGLE_UNIT()
);
#38537=SHAPE_DEFINITION_REPRESENTATION(#38550,#38579);
#38550=PRODUCT_DEFINITION_SHAPE('',$,#38593);
#38579=SHAPE_REPRESENTATION('',(#18641),#38519);
#38588=PRODUCT_DEFINITION_CONTEXT('part definition',#38629,'design');
#38593=PRODUCT_DEFINITION('2026-10-20-13-39-08-151',
'04_Central_Spindle_D10_M6',#38606,#38588);
#38606=PRODUCT_DEFINITION_FORMATION('',$,#38635);
#38629=APPLICATION_CONTEXT(
'Core Data for Automotive Mechanical Design Process');
#38630=PRODUCT_CONTEXT('part definition',#38629,'mechanical');
#38635=PRODUCT('2026-10-20-13-39-08-151','04_Central_Spindle_D10_M6',$,
(#38630));
#38686=COLOUR_RGB('Light Blue',0.38,0.62,0.78);
#38687=FILL_AREA_STYLE_COLOUR('',#38686);
#38688=FILL_AREA_STYLE('',(#38687));
#38689=SURFACE_STYLE_FILL_AREA(#38688);
#38690=SURFACE_SIDE_STYLE('',(#38689));
#38691=SURFACE_STYLE_USAGE(.BOTH.,#38690);
#38692=PRESENTATION_STYLE_ASSIGNMENT((#38691));
ENDSEC;
END-ISO-10303-21;
